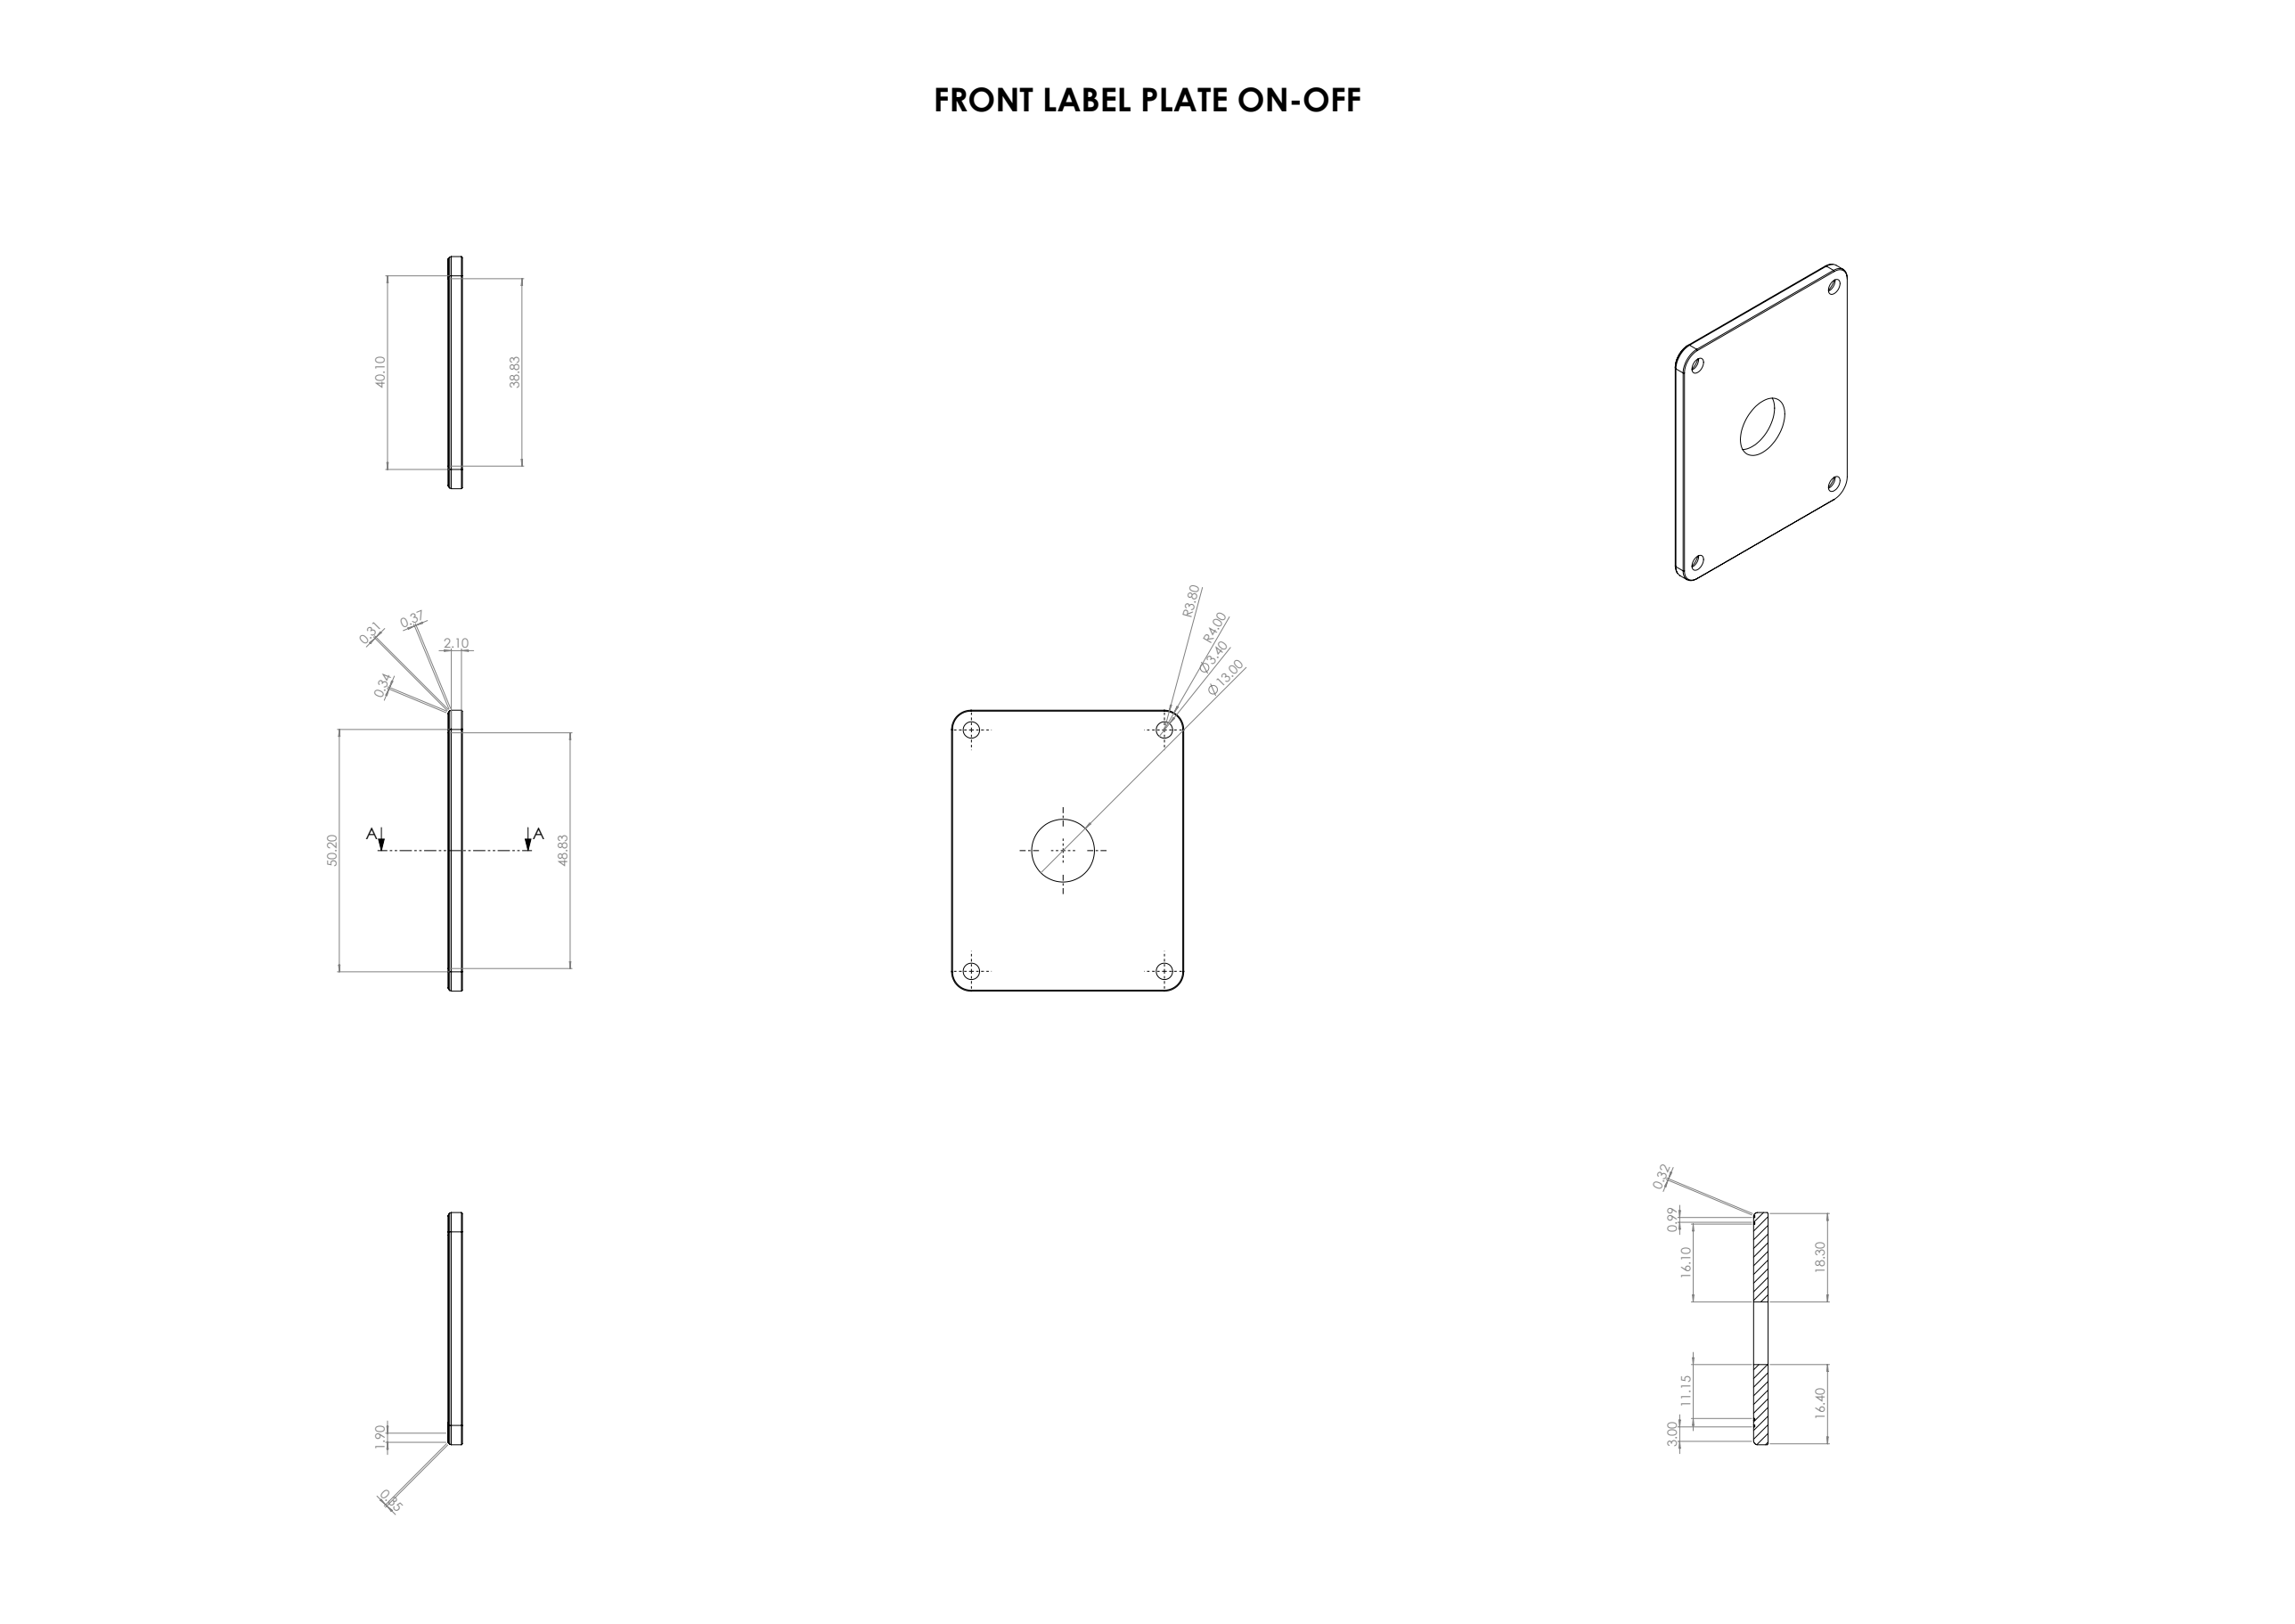
ISO-10303-21;
HEADER;
/* Generated by software containing ST-Developer
 * from STEP Tools, Inc. (www.steptools.com) 
 */

FILE_DESCRIPTION(
/* description */ (''),
/* implementation_level */ '2;1');

FILE_NAME(
/* name */ '06_Front_Label_Plate_ON-OFF.step',
/* time_stamp */ '2026-10-21T01:59:45-07:00',
/* author */ (''),
/* organization */ (''),
/* preprocessor_version */ 'ST-DEVELOPER v20.2',
/* originating_system */ 'Autodesk Translation Framework v15.15.0.0',
/* authorisation */ '');

FILE_SCHEMA (('AUTOMOTIVE_DESIGN { 1 0 10303 214 3 1 1 }'));
ENDSEC;

DATA;
#10=MECHANICAL_DESIGN_GEOMETRIC_PRESENTATION_REPRESENTATION('',(#465),#18281);
#107=(
BOUNDED_CURVE()
B_SPLINE_CURVE(2,(#12695,#12696,#12697),.UNSPECIFIED.,.F.,.F.)
B_SPLINE_CURVE_WITH_KNOTS((3,3),(0.,0.110982483350979),.UNSPECIFIED.)
CURVE()
GEOMETRIC_REPRESENTATION_ITEM()
RATIONAL_B_SPLINE_CURVE((1.,1.,1.))
REPRESENTATION_ITEM('')
);
#108=(
BOUNDED_CURVE()
B_SPLINE_CURVE(2,(#12710,#12711,#12712),.UNSPECIFIED.,.F.,.F.)
B_SPLINE_CURVE_WITH_KNOTS((3,3),(0.058586025044114,0.117172050088227),
 .UNSPECIFIED.)
CURVE()
GEOMETRIC_REPRESENTATION_ITEM()
RATIONAL_B_SPLINE_CURVE((1.,1.,1.))
REPRESENTATION_ITEM('')
);
#109=(
BOUNDED_CURVE()
B_SPLINE_CURVE(2,(#12739,#12740,#12741),.UNSPECIFIED.,.F.,.F.)
B_SPLINE_CURVE_WITH_KNOTS((3,3),(0.,0.0585860250441136),.UNSPECIFIED.)
CURVE()
GEOMETRIC_REPRESENTATION_ITEM()
RATIONAL_B_SPLINE_CURVE((1.,1.,1.))
REPRESENTATION_ITEM('')
);
#110=(
BOUNDED_CURVE()
B_SPLINE_CURVE(2,(#12754,#12755,#12756),.UNSPECIFIED.,.F.,.F.)
B_SPLINE_CURVE_WITH_KNOTS((3,3),(0.0909175021833372,0.201899986183551),
 .UNSPECIFIED.)
CURVE()
GEOMETRIC_REPRESENTATION_ITEM()
RATIONAL_B_SPLINE_CURVE((1.,1.,1.))
REPRESENTATION_ITEM('')
);
#111=(
BOUNDED_CURVE()
B_SPLINE_CURVE(2,(#12765,#12766,#12767),.UNSPECIFIED.,.F.,.F.)
B_SPLINE_CURVE_WITH_KNOTS((3,3),(0.0485753412182672,0.117172050088219),
 .UNSPECIFIED.)
CURVE()
GEOMETRIC_REPRESENTATION_ITEM()
RATIONAL_B_SPLINE_CURVE((1.,1.,1.))
REPRESENTATION_ITEM('')
);
#112=(
BOUNDED_CURVE()
B_SPLINE_CURVE(2,(#12779,#12780,#12781),.UNSPECIFIED.,.F.,.F.)
B_SPLINE_CURVE_WITH_KNOTS((3,3),(0.0585860250445827,0.117172050088221),
 .UNSPECIFIED.)
CURVE()
GEOMETRIC_REPRESENTATION_ITEM()
RATIONAL_B_SPLINE_CURVE((1.,1.,1.))
REPRESENTATION_ITEM('')
);
#113=(
BOUNDED_CURVE()
B_SPLINE_CURVE(2,(#12785,#12786,#12787),.UNSPECIFIED.,.F.,.F.)
B_SPLINE_CURVE_WITH_KNOTS((3,3),(0.,0.068596708869952),.UNSPECIFIED.)
CURVE()
GEOMETRIC_REPRESENTATION_ITEM()
RATIONAL_B_SPLINE_CURVE((1.,1.,1.))
REPRESENTATION_ITEM('')
);
#114=(
BOUNDED_CURVE()
B_SPLINE_CURVE(2,(#12799,#12800,#12801),.UNSPECIFIED.,.F.,.F.)
B_SPLINE_CURVE_WITH_KNOTS((3,3),(0.0485753412182676,0.0585860250445827),
 .UNSPECIFIED.)
CURVE()
GEOMETRIC_REPRESENTATION_ITEM()
RATIONAL_B_SPLINE_CURVE((1.,1.,1.))
REPRESENTATION_ITEM('')
);
#115=(
BOUNDED_CURVE()
B_SPLINE_CURVE(2,(#13088,#13089,#13090),.UNSPECIFIED.,.F.,.F.)
B_SPLINE_CURVE_WITH_KNOTS((3,3),(0.058586025043638,0.0685967088699541),
 .UNSPECIFIED.)
CURVE()
GEOMETRIC_REPRESENTATION_ITEM()
RATIONAL_B_SPLINE_CURVE((1.,1.,1.))
REPRESENTATION_ITEM('')
);
#116=(
BOUNDED_CURVE()
B_SPLINE_CURVE(2,(#13101,#13102,#13103),.UNSPECIFIED.,.F.,.F.)
B_SPLINE_CURVE_WITH_KNOTS((3,3),(0.,0.058586025043638),.UNSPECIFIED.)
CURVE()
GEOMETRIC_REPRESENTATION_ITEM()
RATIONAL_B_SPLINE_CURVE((1.,1.,1.))
REPRESENTATION_ITEM('')
);
#143=B_SPLINE_SURFACE_WITH_KNOTS('',2,1,((#12638,#12639),(#12640,#12641),
(#12642,#12643),(#12644,#12645),(#12646,#12647),(#12648,#12649),(#12650,
#12651)),.UNSPECIFIED.,.F.,.F.,.F.,(3,2,2,3),(2,2),(-1.09408743911249,0.,
1.,1.84668421503224),(-0.0908822509939087,0.140882250993909),
 .UNSPECIFIED.);
#144=B_SPLINE_SURFACE_WITH_KNOTS('',2,1,((#13225,#13226),(#13227,#13228),
(#13229,#13230),(#13231,#13232),(#13233,#13234),(#13235,#13236),(#13237,
#13238)),.UNSPECIFIED.,.F.,.F.,.F.,(3,2,2,3),(2,2),(-0.763868143299771,
0.,1.,1.96021762995607),(-0.090882250993909,0.140882250993909),
 .UNSPECIFIED.);
#145=B_SPLINE_SURFACE_WITH_KNOTS('',2,1,((#13240,#13241),(#13242,#13243),
(#13244,#13245)),.UNSPECIFIED.,.F.,.F.,.F.,(3,3),(2,2),(0.,1.),(0.,0.025),
 .UNSPECIFIED.);
#146=B_SPLINE_SURFACE_WITH_KNOTS('',2,1,((#13247,#13248),(#13249,#13250),
(#13251,#13252)),.UNSPECIFIED.,.F.,.F.,.F.,(3,3),(2,2),(0.,1.),(0.,0.025),
 .UNSPECIFIED.);
#147=B_SPLINE_SURFACE_WITH_KNOTS('',2,1,((#13254,#13255),(#13256,#13257),
(#13258,#13259)),.UNSPECIFIED.,.F.,.F.,.F.,(3,3),(2,2),(0.,1.),(0.,0.025),
 .UNSPECIFIED.);
#148=B_SPLINE_SURFACE_WITH_KNOTS('',2,1,((#13261,#13262),(#13263,#13264),
(#13265,#13266)),.UNSPECIFIED.,.F.,.F.,.F.,(3,3),(2,2),(0.,1.),(0.,0.025),
 .UNSPECIFIED.);
#149=B_SPLINE_SURFACE_WITH_KNOTS('',2,1,((#13268,#13269),(#13270,#13271),
(#13272,#13273)),.UNSPECIFIED.,.F.,.F.,.F.,(3,3),(2,2),(0.,1.),(0.,0.025),
 .UNSPECIFIED.);
#150=B_SPLINE_SURFACE_WITH_KNOTS('',2,1,((#13356,#13357),(#13358,#13359),
(#13360,#13361)),.UNSPECIFIED.,.F.,.F.,.F.,(3,3),(2,2),(0.,1.),(0.,0.025),
 .UNSPECIFIED.);
#151=B_SPLINE_SURFACE_WITH_KNOTS('',2,1,((#13369,#13370),(#13371,#13372),
(#13373,#13374)),.UNSPECIFIED.,.F.,.F.,.F.,(3,3),(2,2),(0.,1.),(0.,0.025),
 .UNSPECIFIED.);
#152=B_SPLINE_SURFACE_WITH_KNOTS('',2,1,((#13380,#13381),(#13382,#13383),
(#13384,#13385)),.UNSPECIFIED.,.F.,.F.,.F.,(3,3),(2,2),(0.,1.),(0.,0.025),
 .UNSPECIFIED.);
#153=B_SPLINE_SURFACE_WITH_KNOTS('',2,1,((#13391,#13392),(#13393,#13394),
(#13395,#13396)),.UNSPECIFIED.,.F.,.F.,.F.,(3,3),(2,2),(0.,1.),(0.,0.025),
 .UNSPECIFIED.);
#154=B_SPLINE_SURFACE_WITH_KNOTS('',2,1,((#13402,#13403),(#13404,#13405),
(#13406,#13407)),.UNSPECIFIED.,.F.,.F.,.F.,(3,3),(2,2),(0.,1.),(0.,0.025),
 .UNSPECIFIED.);
#155=B_SPLINE_SURFACE_WITH_KNOTS('',2,1,((#13413,#13414),(#13415,#13416),
(#13417,#13418)),.UNSPECIFIED.,.F.,.F.,.F.,(3,3),(2,2),(0.,1.),(0.,0.025),
 .UNSPECIFIED.);
#156=B_SPLINE_SURFACE_WITH_KNOTS('',2,1,((#13424,#13425),(#13426,#13427),
(#13428,#13429)),.UNSPECIFIED.,.F.,.F.,.F.,(3,3),(2,2),(0.,1.),(0.,0.025),
 .UNSPECIFIED.);
#157=B_SPLINE_SURFACE_WITH_KNOTS('',2,1,((#13435,#13436),(#13437,#13438),
(#13439,#13440)),.UNSPECIFIED.,.F.,.F.,.F.,(3,3),(2,2),(0.,1.),(0.,0.025),
 .UNSPECIFIED.);
#158=B_SPLINE_SURFACE_WITH_KNOTS('',2,1,((#13446,#13447),(#13448,#13449),
(#13450,#13451)),.UNSPECIFIED.,.F.,.F.,.F.,(3,3),(2,2),(0.,1.),(0.,0.025),
 .UNSPECIFIED.);
#159=B_SPLINE_SURFACE_WITH_KNOTS('',2,1,((#13457,#13458),(#13459,#13460),
(#13461,#13462)),.UNSPECIFIED.,.F.,.F.,.F.,(3,3),(2,2),(0.,1.),(0.,0.025),
 .UNSPECIFIED.);
#160=B_SPLINE_SURFACE_WITH_KNOTS('',2,1,((#13468,#13469),(#13470,#13471),
(#13472,#13473)),.UNSPECIFIED.,.F.,.F.,.F.,(3,3),(2,2),(0.,1.),(0.,0.025),
 .UNSPECIFIED.);
#161=B_SPLINE_SURFACE_WITH_KNOTS('',2,1,((#13519,#13520),(#13521,#13522),
(#13523,#13524)),.UNSPECIFIED.,.F.,.F.,.F.,(3,3),(2,2),(0.,1.),(0.,0.025),
 .UNSPECIFIED.);
#162=B_SPLINE_SURFACE_WITH_KNOTS('',2,1,((#13532,#13533),(#13534,#13535),
(#13536,#13537)),.UNSPECIFIED.,.F.,.F.,.F.,(3,3),(2,2),(0.,1.),(0.,0.025),
 .UNSPECIFIED.);
#163=B_SPLINE_SURFACE_WITH_KNOTS('',2,1,((#13543,#13544),(#13545,#13546),
(#13547,#13548)),.UNSPECIFIED.,.F.,.F.,.F.,(3,3),(2,2),(0.,1.),(0.,0.025),
 .UNSPECIFIED.);
#164=B_SPLINE_SURFACE_WITH_KNOTS('',2,1,((#13554,#13555),(#13556,#13557),
(#13558,#13559)),.UNSPECIFIED.,.F.,.F.,.F.,(3,3),(2,2),(0.,1.),(0.,0.025),
 .UNSPECIFIED.);
#165=B_SPLINE_SURFACE_WITH_KNOTS('',2,1,((#13565,#13566),(#13567,#13568),
(#13569,#13570)),.UNSPECIFIED.,.F.,.F.,.F.,(3,3),(2,2),(0.,1.),(0.,0.025),
 .UNSPECIFIED.);
#166=B_SPLINE_SURFACE_WITH_KNOTS('',2,1,((#13576,#13577),(#13578,#13579),
(#13580,#13581)),.UNSPECIFIED.,.F.,.F.,.F.,(3,3),(2,2),(0.,1.),(0.,0.025),
 .UNSPECIFIED.);
#167=B_SPLINE_SURFACE_WITH_KNOTS('',2,1,((#13587,#13588),(#13589,#13590),
(#13591,#13592)),.UNSPECIFIED.,.F.,.F.,.F.,(3,3),(2,2),(0.,1.),(0.,0.025),
 .UNSPECIFIED.);
#168=B_SPLINE_SURFACE_WITH_KNOTS('',2,1,((#13598,#13599),(#13600,#13601),
(#13602,#13603)),.UNSPECIFIED.,.F.,.F.,.F.,(3,3),(2,2),(0.,1.),(0.,0.025),
 .UNSPECIFIED.);
#169=B_SPLINE_SURFACE_WITH_KNOTS('',2,1,((#13609,#13610),(#13611,#13612),
(#13613,#13614)),.UNSPECIFIED.,.F.,.F.,.F.,(3,3),(2,2),(0.,1.),(0.,0.025),
 .UNSPECIFIED.);
#170=B_SPLINE_SURFACE_WITH_KNOTS('',2,1,((#13620,#13621),(#13622,#13623),
(#13624,#13625)),.UNSPECIFIED.,.F.,.F.,.F.,(3,3),(2,2),(0.,1.),(0.,0.025),
 .UNSPECIFIED.);
#171=B_SPLINE_SURFACE_WITH_KNOTS('',2,1,((#13631,#13632),(#13633,#13634),
(#13635,#13636)),.UNSPECIFIED.,.F.,.F.,.F.,(3,3),(2,2),(0.,1.),(0.,0.025),
 .UNSPECIFIED.);
#172=B_SPLINE_SURFACE_WITH_KNOTS('',2,1,((#13682,#13683),(#13684,#13685),
(#13686,#13687)),.UNSPECIFIED.,.F.,.F.,.F.,(3,3),(2,2),(0.,1.),(0.,0.025),
 .UNSPECIFIED.);
#173=B_SPLINE_SURFACE_WITH_KNOTS('',2,1,((#13695,#13696),(#13697,#13698),
(#13699,#13700)),.UNSPECIFIED.,.F.,.F.,.F.,(3,3),(2,2),(0.,1.),(0.,0.025),
 .UNSPECIFIED.);
#174=B_SPLINE_SURFACE_WITH_KNOTS('',2,1,((#13706,#13707),(#13708,#13709),
(#13710,#13711)),.UNSPECIFIED.,.F.,.F.,.F.,(3,3),(2,2),(0.,1.),(0.,0.025),
 .UNSPECIFIED.);
#175=B_SPLINE_SURFACE_WITH_KNOTS('',2,1,((#13717,#13718),(#13719,#13720),
(#13721,#13722)),.UNSPECIFIED.,.F.,.F.,.F.,(3,3),(2,2),(0.,1.),(0.,0.025),
 .UNSPECIFIED.);
#176=B_SPLINE_SURFACE_WITH_KNOTS('',2,1,((#13728,#13729),(#13730,#13731),
(#13732,#13733)),.UNSPECIFIED.,.F.,.F.,.F.,(3,3),(2,2),(0.,1.),(0.,0.025),
 .UNSPECIFIED.);
#177=B_SPLINE_SURFACE_WITH_KNOTS('',2,1,((#13739,#13740),(#13741,#13742),
(#13743,#13744)),.UNSPECIFIED.,.F.,.F.,.F.,(3,3),(2,2),(0.,1.),(0.,0.025),
 .UNSPECIFIED.);
#178=B_SPLINE_SURFACE_WITH_KNOTS('',2,1,((#13750,#13751),(#13752,#13753),
(#13754,#13755)),.UNSPECIFIED.,.F.,.F.,.F.,(3,3),(2,2),(0.,1.),(0.,0.025),
 .UNSPECIFIED.);
#179=B_SPLINE_SURFACE_WITH_KNOTS('',2,1,((#13761,#13762),(#13763,#13764),
(#13765,#13766)),.UNSPECIFIED.,.F.,.F.,.F.,(3,3),(2,2),(0.,1.),(0.,0.025),
 .UNSPECIFIED.);
#180=B_SPLINE_SURFACE_WITH_KNOTS('',2,1,((#13772,#13773),(#13774,#13775),
(#13776,#13777)),.UNSPECIFIED.,.F.,.F.,.F.,(3,3),(2,2),(0.,1.),(0.,0.025),
 .UNSPECIFIED.);
#181=B_SPLINE_SURFACE_WITH_KNOTS('',2,1,((#13783,#13784),(#13785,#13786),
(#13787,#13788)),.UNSPECIFIED.,.F.,.F.,.F.,(3,3),(2,2),(0.,1.),(0.,0.025),
 .UNSPECIFIED.);
#182=B_SPLINE_SURFACE_WITH_KNOTS('',2,1,((#13794,#13795),(#13796,#13797),
(#13798,#13799)),.UNSPECIFIED.,.F.,.F.,.F.,(3,3),(2,2),(0.,1.),(0.,0.025),
 .UNSPECIFIED.);
#188=B_SPLINE_CURVE_WITH_KNOTS('',3,(#12551,#12552,#12553,#12554),
 .UNSPECIFIED.,.F.,.F.,(4,4),(-0.0416286806186443,-0.039090786429231),
 .UNSPECIFIED.);
#189=B_SPLINE_CURVE_WITH_KNOTS('',3,(#12563,#12564,#12565,#12566),
 .UNSPECIFIED.,.F.,.F.,(4,4),(-0.00358674747543116,-0.00105074276589837),
 .UNSPECIFIED.);
#190=B_SPLINE_CURVE_WITH_KNOTS('',3,(#12609,#12610,#12611,#12612,#12613,
#12614,#12615),.UNSPECIFIED.,.F.,.F.,(4,3,4),(0.,0.0165311745375961,0.035733654742842),
 .UNSPECIFIED.);
#191=B_SPLINE_CURVE_WITH_KNOTS('',3,(#12616,#12617,#12618,#12619,#12620,
#12621,#12622),.UNSPECIFIED.,.F.,.F.,(4,3,4),(0.093322390013544,0.111401256244007,
0.119257131462378),.UNSPECIFIED.);
#192=B_SPLINE_CURVE_WITH_KNOTS('',3,(#12625,#12626,#12627,#12628,#12629,
#12630,#12631),.UNSPECIFIED.,.F.,.F.,(4,3,4),(0.107846162587432,0.120934849613304,
0.1266096642358),.UNSPECIFIED.);
#193=B_SPLINE_CURVE_WITH_KNOTS('',3,(#12633,#12634,#12635,#12636),
 .UNSPECIFIED.,.F.,.F.,(4,4),(0.,0.0156100092084493),.UNSPECIFIED.);
#194=B_SPLINE_CURVE_WITH_KNOTS('',3,(#12653,#12654,#12655,#12656),
 .UNSPECIFIED.,.F.,.F.,(4,4),(-0.159704010702857,-0.0871316914258202),
 .UNSPECIFIED.);
#195=B_SPLINE_CURVE_WITH_KNOTS('',2,(#12658,#12659,#12660),
 .UNSPECIFIED.,.F.,.F.,(3,3),(0.626600308945203,1.),.UNSPECIFIED.);
#196=B_SPLINE_CURVE_WITH_KNOTS('',2,(#12664,#12665,#12666),
 .UNSPECIFIED.,.F.,.F.,(3,3),(0.930285828630975,1.),.UNSPECIFIED.);
#197=B_SPLINE_CURVE_WITH_KNOTS('',3,(#12667,#12668,#12669,#12670,#12671,
#12672,#12673),.UNSPECIFIED.,.F.,.F.,(4,3,4),(-0.0373027797814653,-0.0240644534710859,
0.),.UNSPECIFIED.);
#198=B_SPLINE_CURVE_WITH_KNOTS('',3,(#12676,#12677,#12678,#12679,#12680,
#12681,#12682,#12683,#12684,#12685),.UNSPECIFIED.,.F.,.F.,(4,3,3,4),(-0.19290526608905,
-0.149564698200622,-0.106837983631372,-0.0956446006455143),
 .UNSPECIFIED.);
#199=B_SPLINE_CURVE_WITH_KNOTS('',3,(#12699,#12700,#12701,#12702,#12703,
#12704,#12705,#12706,#12707,#12708),.UNSPECIFIED.,.F.,.F.,(4,2,2,2,4),(0.00995060155970214,
0.127861262644591,0.255722525289182,0.384625287958343,0.513528050627505),
 .UNSPECIFIED.);
#200=B_SPLINE_CURVE_WITH_KNOTS('',3,(#12743,#12744,#12745,#12746,#12747,
#12748,#12749,#12750,#12751,#12752),.UNSPECIFIED.,.F.,.F.,(4,2,2,2,4),(1.52050309692962,
1.64940585959878,1.77830862226794,1.90616988491253,2.02408054599742),
 .UNSPECIFIED.);
#201=B_SPLINE_CURVE_WITH_KNOTS('',3,(#12789,#12790,#12791,#12792,#12793,
#12794,#12795,#12796,#12797,#12798),.UNSPECIFIED.,.F.,.F.,(4,2,2,2,4),(0.518398684879072,
0.638089519791373,0.767732342509753,0.897375165228133,1.01706600014044),
 .UNSPECIFIED.);
#202=B_SPLINE_CURVE_WITH_KNOTS('',2,(#12813,#12814,#12815),
 .UNSPECIFIED.,.F.,.F.,(3,3),(0.,1.),.UNSPECIFIED.);
#203=B_SPLINE_CURVE_WITH_KNOTS('',2,(#12817,#12818,#12819),
 .UNSPECIFIED.,.F.,.F.,(3,3),(0.,1.),.UNSPECIFIED.);
#204=B_SPLINE_CURVE_WITH_KNOTS('',2,(#12821,#12822,#12823),
 .UNSPECIFIED.,.F.,.F.,(3,3),(0.,1.),.UNSPECIFIED.);
#205=B_SPLINE_CURVE_WITH_KNOTS('',2,(#12825,#12826,#12827),
 .UNSPECIFIED.,.F.,.F.,(3,3),(0.,1.),.UNSPECIFIED.);
#206=B_SPLINE_CURVE_WITH_KNOTS('',2,(#12829,#12830,#12831),
 .UNSPECIFIED.,.F.,.F.,(3,3),(0.,1.),.UNSPECIFIED.);
#207=B_SPLINE_CURVE_WITH_KNOTS('',2,(#12832,#12833,#12834),
 .UNSPECIFIED.,.F.,.F.,(3,3),(0.,0.31406597767443),.UNSPECIFIED.);
#208=B_SPLINE_CURVE_WITH_KNOTS('',2,(#12906,#12907,#12908),
 .UNSPECIFIED.,.F.,.F.,(3,3),(0.,1.),.UNSPECIFIED.);
#209=B_SPLINE_CURVE_WITH_KNOTS('',2,(#12910,#12911,#12912),
 .UNSPECIFIED.,.F.,.F.,(3,3),(0.,1.),.UNSPECIFIED.);
#210=B_SPLINE_CURVE_WITH_KNOTS('',2,(#12914,#12915,#12916),
 .UNSPECIFIED.,.F.,.F.,(3,3),(0.,1.),.UNSPECIFIED.);
#211=B_SPLINE_CURVE_WITH_KNOTS('',2,(#12918,#12919,#12920),
 .UNSPECIFIED.,.F.,.F.,(3,3),(0.,1.),.UNSPECIFIED.);
#212=B_SPLINE_CURVE_WITH_KNOTS('',2,(#12922,#12923,#12924),
 .UNSPECIFIED.,.F.,.F.,(3,3),(0.,1.),.UNSPECIFIED.);
#213=B_SPLINE_CURVE_WITH_KNOTS('',2,(#12926,#12927,#12928),
 .UNSPECIFIED.,.F.,.F.,(3,3),(0.,1.),.UNSPECIFIED.);
#214=B_SPLINE_CURVE_WITH_KNOTS('',2,(#12930,#12931,#12932),
 .UNSPECIFIED.,.F.,.F.,(3,3),(0.,1.),.UNSPECIFIED.);
#215=B_SPLINE_CURVE_WITH_KNOTS('',2,(#12934,#12935,#12936),
 .UNSPECIFIED.,.F.,.F.,(3,3),(0.,1.),.UNSPECIFIED.);
#216=B_SPLINE_CURVE_WITH_KNOTS('',2,(#12938,#12939,#12940),
 .UNSPECIFIED.,.F.,.F.,(3,3),(0.,1.),.UNSPECIFIED.);
#217=B_SPLINE_CURVE_WITH_KNOTS('',2,(#12942,#12943,#12944),
 .UNSPECIFIED.,.F.,.F.,(3,3),(0.,1.),.UNSPECIFIED.);
#218=B_SPLINE_CURVE_WITH_KNOTS('',2,(#12945,#12946,#12947),
 .UNSPECIFIED.,.F.,.F.,(3,3),(0.,1.),.UNSPECIFIED.);
#219=B_SPLINE_CURVE_WITH_KNOTS('',2,(#12970,#12971,#12972),
 .UNSPECIFIED.,.F.,.F.,(3,3),(0.,1.),.UNSPECIFIED.);
#220=B_SPLINE_CURVE_WITH_KNOTS('',2,(#12974,#12975,#12976),
 .UNSPECIFIED.,.F.,.F.,(3,3),(0.,1.),.UNSPECIFIED.);
#221=B_SPLINE_CURVE_WITH_KNOTS('',2,(#12978,#12979,#12980),
 .UNSPECIFIED.,.F.,.F.,(3,3),(0.,1.),.UNSPECIFIED.);
#222=B_SPLINE_CURVE_WITH_KNOTS('',2,(#12982,#12983,#12984),
 .UNSPECIFIED.,.F.,.F.,(3,3),(0.,1.),.UNSPECIFIED.);
#223=B_SPLINE_CURVE_WITH_KNOTS('',2,(#12986,#12987,#12988),
 .UNSPECIFIED.,.F.,.F.,(3,3),(0.,1.),.UNSPECIFIED.);
#224=B_SPLINE_CURVE_WITH_KNOTS('',2,(#12990,#12991,#12992),
 .UNSPECIFIED.,.F.,.F.,(3,3),(0.,1.),.UNSPECIFIED.);
#225=B_SPLINE_CURVE_WITH_KNOTS('',2,(#12994,#12995,#12996),
 .UNSPECIFIED.,.F.,.F.,(3,3),(0.,1.),.UNSPECIFIED.);
#226=B_SPLINE_CURVE_WITH_KNOTS('',2,(#12998,#12999,#13000),
 .UNSPECIFIED.,.F.,.F.,(3,3),(0.,1.),.UNSPECIFIED.);
#227=B_SPLINE_CURVE_WITH_KNOTS('',2,(#13002,#13003,#13004),
 .UNSPECIFIED.,.F.,.F.,(3,3),(0.,1.),.UNSPECIFIED.);
#228=B_SPLINE_CURVE_WITH_KNOTS('',2,(#13006,#13007,#13008),
 .UNSPECIFIED.,.F.,.F.,(3,3),(0.,1.),.UNSPECIFIED.);
#229=B_SPLINE_CURVE_WITH_KNOTS('',2,(#13009,#13010,#13011),
 .UNSPECIFIED.,.F.,.F.,(3,3),(0.,1.),.UNSPECIFIED.);
#230=B_SPLINE_CURVE_WITH_KNOTS('',2,(#13016,#13017,#13018),
 .UNSPECIFIED.,.F.,.F.,(3,3),(0.,1.),.UNSPECIFIED.);
#231=B_SPLINE_CURVE_WITH_KNOTS('',2,(#13020,#13021,#13022),
 .UNSPECIFIED.,.F.,.F.,(3,3),(0.,1.),.UNSPECIFIED.);
#232=B_SPLINE_CURVE_WITH_KNOTS('',2,(#13024,#13025,#13026),
 .UNSPECIFIED.,.F.,.F.,(3,3),(0.,1.),.UNSPECIFIED.);
#233=B_SPLINE_CURVE_WITH_KNOTS('',2,(#13028,#13029,#13030),
 .UNSPECIFIED.,.F.,.F.,(3,3),(0.,1.),.UNSPECIFIED.);
#234=B_SPLINE_CURVE_WITH_KNOTS('',2,(#13032,#13033,#13034),
 .UNSPECIFIED.,.F.,.F.,(3,3),(0.,1.),.UNSPECIFIED.);
#235=B_SPLINE_CURVE_WITH_KNOTS('',2,(#13036,#13037,#13038),
 .UNSPECIFIED.,.F.,.F.,(3,3),(0.,1.),.UNSPECIFIED.);
#236=B_SPLINE_CURVE_WITH_KNOTS('',2,(#13040,#13041,#13042),
 .UNSPECIFIED.,.F.,.F.,(3,3),(0.,1.),.UNSPECIFIED.);
#237=B_SPLINE_CURVE_WITH_KNOTS('',2,(#13044,#13045,#13046),
 .UNSPECIFIED.,.F.,.F.,(3,3),(0.,1.),.UNSPECIFIED.);
#238=B_SPLINE_CURVE_WITH_KNOTS('',2,(#13048,#13049,#13050),
 .UNSPECIFIED.,.F.,.F.,(3,3),(0.,1.),.UNSPECIFIED.);
#239=B_SPLINE_CURVE_WITH_KNOTS('',2,(#13052,#13053,#13054),
 .UNSPECIFIED.,.F.,.F.,(3,3),(0.,1.),.UNSPECIFIED.);
#240=B_SPLINE_CURVE_WITH_KNOTS('',2,(#13055,#13056,#13057),
 .UNSPECIFIED.,.F.,.F.,(3,3),(0.,1.),.UNSPECIFIED.);
#241=B_SPLINE_CURVE_WITH_KNOTS('',3,(#13091,#13092,#13093,#13094,#13095,
#13096,#13097,#13098,#13099,#13100),.UNSPECIFIED.,.F.,.F.,(4,2,2,2,4),(1.01688813186998,
1.13657896678228,1.26622178950066,1.39586461221904,1.51555544713135),
 .UNSPECIFIED.);
#242=B_SPLINE_CURVE_WITH_KNOTS('',2,(#13149,#13150,#13151),
 .UNSPECIFIED.,.F.,.F.,(3,3),(0.,0.369411589751801),.UNSPECIFIED.);
#243=B_SPLINE_CURVE_WITH_KNOTS('',2,(#13153,#13154,#13155),
 .UNSPECIFIED.,.F.,.F.,(3,3),(0.,1.),.UNSPECIFIED.);
#244=B_SPLINE_CURVE_WITH_KNOTS('',2,(#13157,#13158,#13159),
 .UNSPECIFIED.,.F.,.F.,(3,3),(0.,1.),.UNSPECIFIED.);
#245=B_SPLINE_CURVE_WITH_KNOTS('',2,(#13161,#13162,#13163),
 .UNSPECIFIED.,.F.,.F.,(3,3),(0.,1.),.UNSPECIFIED.);
#246=B_SPLINE_CURVE_WITH_KNOTS('',2,(#13165,#13166,#13167),
 .UNSPECIFIED.,.F.,.F.,(3,3),(0.,1.),.UNSPECIFIED.);
#247=B_SPLINE_CURVE_WITH_KNOTS('',2,(#13168,#13169,#13170),
 .UNSPECIFIED.,.F.,.F.,(3,3),(0.,1.),.UNSPECIFIED.);
#248=B_SPLINE_CURVE_WITH_KNOTS('',2,(#13365,#13366,#13367),
 .UNSPECIFIED.,.F.,.F.,(3,3),(0.,1.),.UNSPECIFIED.);
#249=B_SPLINE_CURVE_WITH_KNOTS('',2,(#13377,#13378,#13379),
 .UNSPECIFIED.,.F.,.F.,(3,3),(0.,1.),.UNSPECIFIED.);
#250=B_SPLINE_CURVE_WITH_KNOTS('',2,(#13388,#13389,#13390),
 .UNSPECIFIED.,.F.,.F.,(3,3),(0.,1.),.UNSPECIFIED.);
#251=B_SPLINE_CURVE_WITH_KNOTS('',2,(#13399,#13400,#13401),
 .UNSPECIFIED.,.F.,.F.,(3,3),(0.,1.),.UNSPECIFIED.);
#252=B_SPLINE_CURVE_WITH_KNOTS('',2,(#13410,#13411,#13412),
 .UNSPECIFIED.,.F.,.F.,(3,3),(0.,1.),.UNSPECIFIED.);
#253=B_SPLINE_CURVE_WITH_KNOTS('',2,(#13421,#13422,#13423),
 .UNSPECIFIED.,.F.,.F.,(3,3),(0.,1.),.UNSPECIFIED.);
#254=B_SPLINE_CURVE_WITH_KNOTS('',2,(#13432,#13433,#13434),
 .UNSPECIFIED.,.F.,.F.,(3,3),(0.,1.),.UNSPECIFIED.);
#255=B_SPLINE_CURVE_WITH_KNOTS('',2,(#13443,#13444,#13445),
 .UNSPECIFIED.,.F.,.F.,(3,3),(0.,1.),.UNSPECIFIED.);
#256=B_SPLINE_CURVE_WITH_KNOTS('',2,(#13454,#13455,#13456),
 .UNSPECIFIED.,.F.,.F.,(3,3),(0.,1.),.UNSPECIFIED.);
#257=B_SPLINE_CURVE_WITH_KNOTS('',2,(#13465,#13466,#13467),
 .UNSPECIFIED.,.F.,.F.,(3,3),(0.,1.),.UNSPECIFIED.);
#258=B_SPLINE_CURVE_WITH_KNOTS('',2,(#13474,#13475,#13476),
 .UNSPECIFIED.,.F.,.F.,(3,3),(0.,1.),.UNSPECIFIED.);
#259=B_SPLINE_CURVE_WITH_KNOTS('',2,(#13528,#13529,#13530),
 .UNSPECIFIED.,.F.,.F.,(3,3),(0.,1.),.UNSPECIFIED.);
#260=B_SPLINE_CURVE_WITH_KNOTS('',2,(#13540,#13541,#13542),
 .UNSPECIFIED.,.F.,.F.,(3,3),(0.,1.),.UNSPECIFIED.);
#261=B_SPLINE_CURVE_WITH_KNOTS('',2,(#13551,#13552,#13553),
 .UNSPECIFIED.,.F.,.F.,(3,3),(0.,1.),.UNSPECIFIED.);
#262=B_SPLINE_CURVE_WITH_KNOTS('',2,(#13562,#13563,#13564),
 .UNSPECIFIED.,.F.,.F.,(3,3),(0.,1.),.UNSPECIFIED.);
#263=B_SPLINE_CURVE_WITH_KNOTS('',2,(#13573,#13574,#13575),
 .UNSPECIFIED.,.F.,.F.,(3,3),(0.,1.),.UNSPECIFIED.);
#264=B_SPLINE_CURVE_WITH_KNOTS('',2,(#13584,#13585,#13586),
 .UNSPECIFIED.,.F.,.F.,(3,3),(0.,1.),.UNSPECIFIED.);
#265=B_SPLINE_CURVE_WITH_KNOTS('',2,(#13595,#13596,#13597),
 .UNSPECIFIED.,.F.,.F.,(3,3),(0.,1.),.UNSPECIFIED.);
#266=B_SPLINE_CURVE_WITH_KNOTS('',2,(#13606,#13607,#13608),
 .UNSPECIFIED.,.F.,.F.,(3,3),(0.,1.),.UNSPECIFIED.);
#267=B_SPLINE_CURVE_WITH_KNOTS('',2,(#13617,#13618,#13619),
 .UNSPECIFIED.,.F.,.F.,(3,3),(0.,1.),.UNSPECIFIED.);
#268=B_SPLINE_CURVE_WITH_KNOTS('',2,(#13628,#13629,#13630),
 .UNSPECIFIED.,.F.,.F.,(3,3),(0.,1.),.UNSPECIFIED.);
#269=B_SPLINE_CURVE_WITH_KNOTS('',2,(#13637,#13638,#13639),
 .UNSPECIFIED.,.F.,.F.,(3,3),(0.,1.),.UNSPECIFIED.);
#270=B_SPLINE_CURVE_WITH_KNOTS('',2,(#13691,#13692,#13693),
 .UNSPECIFIED.,.F.,.F.,(3,3),(0.,1.),.UNSPECIFIED.);
#271=B_SPLINE_CURVE_WITH_KNOTS('',2,(#13703,#13704,#13705),
 .UNSPECIFIED.,.F.,.F.,(3,3),(0.,1.),.UNSPECIFIED.);
#272=B_SPLINE_CURVE_WITH_KNOTS('',2,(#13714,#13715,#13716),
 .UNSPECIFIED.,.F.,.F.,(3,3),(0.,1.),.UNSPECIFIED.);
#273=B_SPLINE_CURVE_WITH_KNOTS('',2,(#13725,#13726,#13727),
 .UNSPECIFIED.,.F.,.F.,(3,3),(0.,1.),.UNSPECIFIED.);
#274=B_SPLINE_CURVE_WITH_KNOTS('',2,(#13736,#13737,#13738),
 .UNSPECIFIED.,.F.,.F.,(3,3),(0.,1.),.UNSPECIFIED.);
#275=B_SPLINE_CURVE_WITH_KNOTS('',2,(#13747,#13748,#13749),
 .UNSPECIFIED.,.F.,.F.,(3,3),(0.,1.),.UNSPECIFIED.);
#276=B_SPLINE_CURVE_WITH_KNOTS('',2,(#13758,#13759,#13760),
 .UNSPECIFIED.,.F.,.F.,(3,3),(0.,1.),.UNSPECIFIED.);
#277=B_SPLINE_CURVE_WITH_KNOTS('',2,(#13769,#13770,#13771),
 .UNSPECIFIED.,.F.,.F.,(3,3),(0.,1.),.UNSPECIFIED.);
#278=B_SPLINE_CURVE_WITH_KNOTS('',2,(#13780,#13781,#13782),
 .UNSPECIFIED.,.F.,.F.,(3,3),(0.,1.),.UNSPECIFIED.);
#279=B_SPLINE_CURVE_WITH_KNOTS('',2,(#13791,#13792,#13793),
 .UNSPECIFIED.,.F.,.F.,(3,3),(0.,1.),.UNSPECIFIED.);
#280=B_SPLINE_CURVE_WITH_KNOTS('',2,(#13800,#13801,#13802),
 .UNSPECIFIED.,.F.,.F.,(3,3),(0.,1.),.UNSPECIFIED.);
#368=CONICAL_SURFACE('',#9304,3.9,0.785398163397444);
#369=CONICAL_SURFACE('',#9308,3.9,0.785398163397444);
#370=CONICAL_SURFACE('',#9312,3.9,0.78539816339745);
#371=CONICAL_SURFACE('',#9316,3.9,0.78539816339745);
#372=CONICAL_SURFACE('',#9332,3.92928932188135,0.392699081698714);
#373=CONICAL_SURFACE('',#9335,3.92928932188135,0.392699081698714);
#374=CONICAL_SURFACE('',#9338,3.92928932188135,0.392699081698713);
#375=CONICAL_SURFACE('',#9342,3.92928932188135,0.392699081698724);
#376=CONICAL_SURFACE('',#9346,3.75,0.785398163397449);
#377=CONICAL_SURFACE('',#9349,3.75,0.785398163397447);
#378=CONICAL_SURFACE('',#9354,3.27928932188134,1.17809724509616);
#379=CONICAL_SURFACE('',#9358,3.47071067811865,1.17809724509617);
#380=CONICAL_SURFACE('',#9361,2.475,0.785398163397448);
#381=CONICAL_SURFACE('',#9363,3.27928932188134,1.17809724509616);
#382=CONICAL_SURFACE('',#9367,3.47071067811866,1.17809724509617);
#383=CONICAL_SURFACE('',#9369,2.475,0.785398163397448);
#384=CONICAL_SURFACE('',#9371,3.27928932188134,1.17809724509614);
#385=CONICAL_SURFACE('',#9378,2.475,0.785398163397449);
#386=CONICAL_SURFACE('',#9380,3.27928932188134,1.17809724509614);
#387=CONICAL_SURFACE('',#9382,2.475,0.785398163397449);
#388=CONICAL_SURFACE('',#9388,3.47071067811866,1.17809724509616);
#389=CONICAL_SURFACE('',#9390,3.47071067811866,1.17809724509616);
#390=CONICAL_SURFACE('',#9393,3.75,0.785398163397449);
#391=CONICAL_SURFACE('',#9395,3.75,0.785398163397449);
#439=SHAPE_REPRESENTATION_RELATIONSHIP('SRR','None',#18341,#452);
#452=ADVANCED_BREP_SHAPE_REPRESENTATION('',(#483),#18270);
#465=STYLED_ITEM('',(#18488),#483);
#483=MANIFOLD_SOLID_BREP('Body1',#9087);
#499=CYLINDRICAL_SURFACE('',#9319,4.);
#500=CYLINDRICAL_SURFACE('',#9322,4.);
#501=CYLINDRICAL_SURFACE('',#9462,1.7);
#502=CYLINDRICAL_SURFACE('',#9463,1.7);
#503=CYLINDRICAL_SURFACE('',#9464,1.7);
#504=CYLINDRICAL_SURFACE('',#9465,1.7);
#505=CYLINDRICAL_SURFACE('',#9466,6.5);
#506=CYLINDRICAL_SURFACE('',#9467,4.);
#507=CYLINDRICAL_SURFACE('',#9468,4.);
#585=FACE_BOUND('',#1422,.T.);
#586=FACE_BOUND('',#1423,.T.);
#587=FACE_BOUND('',#1424,.T.);
#588=FACE_BOUND('',#1425,.T.);
#589=FACE_BOUND('',#1426,.T.);
#590=FACE_BOUND('',#1454,.T.);
#591=FACE_BOUND('',#1455,.T.);
#592=FACE_BOUND('',#1456,.T.);
#593=FACE_BOUND('',#1457,.T.);
#594=FACE_BOUND('',#1458,.T.);
#595=FACE_BOUND('',#1459,.T.);
#596=FACE_BOUND('',#1460,.T.);
#597=FACE_BOUND('',#1461,.T.);
#639=CIRCLE('',#9305,4.);
#640=CIRCLE('',#9306,3.8);
#641=CIRCLE('',#9309,4.);
#642=CIRCLE('',#9310,3.8);
#643=CIRCLE('',#9313,4.);
#644=CIRCLE('',#9314,3.8);
#645=CIRCLE('',#9317,4.);
#646=CIRCLE('',#9318,3.8);
#647=CIRCLE('',#9320,4.);
#648=CIRCLE('',#9323,4.);
#649=CIRCLE('',#9326,1.7);
#650=CIRCLE('',#9327,1.7);
#651=CIRCLE('',#9328,1.7);
#652=CIRCLE('',#9329,1.7);
#653=CIRCLE('',#9330,6.5);
#654=CIRCLE('',#9333,3.85857864376269);
#655=CIRCLE('',#9336,3.85857864376269);
#656=CIRCLE('',#9339,3.85857864376269);
#657=CIRCLE('',#9340,4.);
#658=CIRCLE('',#9343,3.85857864376269);
#659=CIRCLE('',#9344,4.);
#660=CIRCLE('',#9347,3.64142135623731);
#661=CIRCLE('',#9350,3.64142135623731);
#662=CIRCLE('',#9355,3.10857864376269);
#663=CIRCLE('',#9356,3.45);
#664=CIRCLE('',#9357,3.45);
#665=CIRCLE('',#9359,3.64142135623731);
#666=CIRCLE('',#9362,1.7);
#667=CIRCLE('',#9364,3.10857864376269);
#668=CIRCLE('',#9365,3.45);
#669=CIRCLE('',#9366,3.45);
#670=CIRCLE('',#9370,1.7);
#671=CIRCLE('',#9372,3.1085786437627);
#672=CIRCLE('',#9373,3.44999999999999);
#673=CIRCLE('',#9376,3.44999999999999);
#674=CIRCLE('',#9377,6.5);
#675=CIRCLE('',#9379,1.7);
#676=CIRCLE('',#9381,3.1085786437627);
#677=CIRCLE('',#9383,1.7);
#678=CIRCLE('',#9391,3.64142135623731);
#881=FACE_OUTER_BOUND('',#1409,.T.);
#882=FACE_OUTER_BOUND('',#1410,.T.);
#883=FACE_OUTER_BOUND('',#1411,.T.);
#884=FACE_OUTER_BOUND('',#1412,.T.);
#885=FACE_OUTER_BOUND('',#1413,.T.);
#886=FACE_OUTER_BOUND('',#1414,.T.);
#887=FACE_OUTER_BOUND('',#1415,.T.);
#888=FACE_OUTER_BOUND('',#1416,.T.);
#889=FACE_OUTER_BOUND('',#1417,.T.);
#890=FACE_OUTER_BOUND('',#1418,.T.);
#891=FACE_OUTER_BOUND('',#1419,.T.);
#892=FACE_OUTER_BOUND('',#1420,.T.);
#893=FACE_OUTER_BOUND('',#1421,.T.);
#894=FACE_OUTER_BOUND('',#1427,.T.);
#895=FACE_OUTER_BOUND('',#1428,.T.);
#896=FACE_OUTER_BOUND('',#1429,.T.);
#897=FACE_OUTER_BOUND('',#1430,.T.);
#898=FACE_OUTER_BOUND('',#1431,.T.);
#899=FACE_OUTER_BOUND('',#1432,.T.);
#900=FACE_OUTER_BOUND('',#1433,.T.);
#901=FACE_OUTER_BOUND('',#1434,.T.);
#902=FACE_OUTER_BOUND('',#1435,.T.);
#903=FACE_OUTER_BOUND('',#1436,.T.);
#904=FACE_OUTER_BOUND('',#1437,.T.);
#905=FACE_OUTER_BOUND('',#1438,.T.);
#906=FACE_OUTER_BOUND('',#1439,.T.);
#907=FACE_OUTER_BOUND('',#1440,.T.);
#908=FACE_OUTER_BOUND('',#1441,.T.);
#909=FACE_OUTER_BOUND('',#1442,.T.);
#910=FACE_OUTER_BOUND('',#1443,.T.);
#911=FACE_OUTER_BOUND('',#1444,.T.);
#912=FACE_OUTER_BOUND('',#1445,.T.);
#913=FACE_OUTER_BOUND('',#1446,.T.);
#914=FACE_OUTER_BOUND('',#1447,.T.);
#915=FACE_OUTER_BOUND('',#1448,.T.);
#916=FACE_OUTER_BOUND('',#1449,.T.);
#917=FACE_OUTER_BOUND('',#1450,.T.);
#918=FACE_OUTER_BOUND('',#1451,.T.);
#919=FACE_OUTER_BOUND('',#1452,.T.);
#920=FACE_OUTER_BOUND('',#1453,.T.);
#921=FACE_OUTER_BOUND('',#1462,.T.);
#922=FACE_OUTER_BOUND('',#1463,.T.);
#923=FACE_OUTER_BOUND('',#1464,.T.);
#924=FACE_OUTER_BOUND('',#1465,.T.);
#925=FACE_OUTER_BOUND('',#1466,.T.);
#926=FACE_OUTER_BOUND('',#1467,.T.);
#927=FACE_OUTER_BOUND('',#1468,.T.);
#928=FACE_OUTER_BOUND('',#1469,.T.);
#929=FACE_OUTER_BOUND('',#1470,.T.);
#930=FACE_OUTER_BOUND('',#1471,.T.);
#931=FACE_OUTER_BOUND('',#1472,.T.);
#932=FACE_OUTER_BOUND('',#1473,.T.);
#933=FACE_OUTER_BOUND('',#1474,.T.);
#934=FACE_OUTER_BOUND('',#1475,.T.);
#935=FACE_OUTER_BOUND('',#1476,.T.);
#936=FACE_OUTER_BOUND('',#1477,.T.);
#937=FACE_OUTER_BOUND('',#1478,.T.);
#938=FACE_OUTER_BOUND('',#1479,.T.);
#939=FACE_OUTER_BOUND('',#1480,.T.);
#940=FACE_OUTER_BOUND('',#1481,.T.);
#941=FACE_OUTER_BOUND('',#1482,.T.);
#942=FACE_OUTER_BOUND('',#1483,.T.);
#943=FACE_OUTER_BOUND('',#1484,.T.);
#944=FACE_OUTER_BOUND('',#1485,.T.);
#945=FACE_OUTER_BOUND('',#1486,.T.);
#946=FACE_OUTER_BOUND('',#1487,.T.);
#947=FACE_OUTER_BOUND('',#1488,.T.);
#948=FACE_OUTER_BOUND('',#1489,.T.);
#949=FACE_OUTER_BOUND('',#1490,.T.);
#950=FACE_OUTER_BOUND('',#1491,.T.);
#951=FACE_OUTER_BOUND('',#1492,.T.);
#952=FACE_OUTER_BOUND('',#1493,.T.);
#953=FACE_OUTER_BOUND('',#1494,.T.);
#954=FACE_OUTER_BOUND('',#1495,.T.);
#955=FACE_OUTER_BOUND('',#1496,.T.);
#956=FACE_OUTER_BOUND('',#1497,.T.);
#957=FACE_OUTER_BOUND('',#1498,.T.);
#958=FACE_OUTER_BOUND('',#1499,.T.);
#959=FACE_OUTER_BOUND('',#1500,.T.);
#960=FACE_OUTER_BOUND('',#1501,.T.);
#961=FACE_OUTER_BOUND('',#1502,.T.);
#962=FACE_OUTER_BOUND('',#1503,.T.);
#963=FACE_OUTER_BOUND('',#1504,.T.);
#964=FACE_OUTER_BOUND('',#1505,.T.);
#965=FACE_OUTER_BOUND('',#1506,.T.);
#966=FACE_OUTER_BOUND('',#1507,.T.);
#967=FACE_OUTER_BOUND('',#1508,.T.);
#968=FACE_OUTER_BOUND('',#1509,.T.);
#969=FACE_OUTER_BOUND('',#1510,.T.);
#970=FACE_OUTER_BOUND('',#1511,.T.);
#971=FACE_OUTER_BOUND('',#1512,.T.);
#972=FACE_OUTER_BOUND('',#1513,.T.);
#973=FACE_OUTER_BOUND('',#1514,.T.);
#974=FACE_OUTER_BOUND('',#1515,.T.);
#975=FACE_OUTER_BOUND('',#1516,.T.);
#976=FACE_OUTER_BOUND('',#1517,.T.);
#977=FACE_OUTER_BOUND('',#1518,.T.);
#978=FACE_OUTER_BOUND('',#1519,.T.);
#979=FACE_OUTER_BOUND('',#1520,.T.);
#980=FACE_OUTER_BOUND('',#1521,.T.);
#981=FACE_OUTER_BOUND('',#1522,.T.);
#982=FACE_OUTER_BOUND('',#1523,.T.);
#983=FACE_OUTER_BOUND('',#1524,.T.);
#984=FACE_OUTER_BOUND('',#1525,.T.);
#985=FACE_OUTER_BOUND('',#1526,.T.);
#986=FACE_OUTER_BOUND('',#1527,.T.);
#987=FACE_OUTER_BOUND('',#1528,.T.);
#988=FACE_OUTER_BOUND('',#1529,.T.);
#989=FACE_OUTER_BOUND('',#1530,.T.);
#990=FACE_OUTER_BOUND('',#1531,.T.);
#991=FACE_OUTER_BOUND('',#1532,.T.);
#992=FACE_OUTER_BOUND('',#1533,.T.);
#993=FACE_OUTER_BOUND('',#1534,.T.);
#994=FACE_OUTER_BOUND('',#1535,.T.);
#995=FACE_OUTER_BOUND('',#1536,.T.);
#996=FACE_OUTER_BOUND('',#1537,.T.);
#997=FACE_OUTER_BOUND('',#1538,.T.);
#998=FACE_OUTER_BOUND('',#1539,.T.);
#999=FACE_OUTER_BOUND('',#1540,.T.);
#1000=FACE_OUTER_BOUND('',#1541,.T.);
#1001=FACE_OUTER_BOUND('',#1542,.T.);
#1002=FACE_OUTER_BOUND('',#1543,.T.);
#1003=FACE_OUTER_BOUND('',#1544,.T.);
#1004=FACE_OUTER_BOUND('',#1545,.T.);
#1005=FACE_OUTER_BOUND('',#1546,.T.);
#1006=FACE_OUTER_BOUND('',#1547,.T.);
#1007=FACE_OUTER_BOUND('',#1548,.T.);
#1008=FACE_OUTER_BOUND('',#1549,.T.);
#1009=FACE_OUTER_BOUND('',#1550,.T.);
#1010=FACE_OUTER_BOUND('',#1551,.T.);
#1011=FACE_OUTER_BOUND('',#1552,.T.);
#1012=FACE_OUTER_BOUND('',#1553,.T.);
#1013=FACE_OUTER_BOUND('',#1554,.T.);
#1014=FACE_OUTER_BOUND('',#1555,.T.);
#1015=FACE_OUTER_BOUND('',#1556,.T.);
#1016=FACE_OUTER_BOUND('',#1557,.T.);
#1017=FACE_OUTER_BOUND('',#1558,.T.);
#1018=FACE_OUTER_BOUND('',#1559,.T.);
#1019=FACE_OUTER_BOUND('',#1560,.T.);
#1020=FACE_OUTER_BOUND('',#1561,.T.);
#1021=FACE_OUTER_BOUND('',#1562,.T.);
#1022=FACE_OUTER_BOUND('',#1563,.T.);
#1023=FACE_OUTER_BOUND('',#1564,.T.);
#1024=FACE_OUTER_BOUND('',#1565,.T.);
#1025=FACE_OUTER_BOUND('',#1566,.T.);
#1026=FACE_OUTER_BOUND('',#1567,.T.);
#1027=FACE_OUTER_BOUND('',#1568,.T.);
#1028=FACE_OUTER_BOUND('',#1569,.T.);
#1029=FACE_OUTER_BOUND('',#1570,.T.);
#1030=FACE_OUTER_BOUND('',#1571,.T.);
#1031=FACE_OUTER_BOUND('',#1572,.T.);
#1032=FACE_OUTER_BOUND('',#1573,.T.);
#1033=FACE_OUTER_BOUND('',#1574,.T.);
#1034=FACE_OUTER_BOUND('',#1575,.T.);
#1035=FACE_OUTER_BOUND('',#1576,.T.);
#1036=FACE_OUTER_BOUND('',#1577,.T.);
#1037=FACE_OUTER_BOUND('',#1578,.T.);
#1038=FACE_OUTER_BOUND('',#1579,.T.);
#1039=FACE_OUTER_BOUND('',#1580,.T.);
#1040=FACE_OUTER_BOUND('',#1581,.T.);
#1041=FACE_OUTER_BOUND('',#1582,.T.);
#1042=FACE_OUTER_BOUND('',#1583,.T.);
#1043=FACE_OUTER_BOUND('',#1584,.T.);
#1044=FACE_OUTER_BOUND('',#1585,.T.);
#1045=FACE_OUTER_BOUND('',#1586,.T.);
#1046=FACE_OUTER_BOUND('',#1587,.T.);
#1047=FACE_OUTER_BOUND('',#1588,.T.);
#1409=EDGE_LOOP('',(#5854,#5855,#5856,#5857));
#1410=EDGE_LOOP('',(#5858,#5859,#5860,#5861));
#1411=EDGE_LOOP('',(#5862,#5863,#5864,#5865));
#1412=EDGE_LOOP('',(#5866,#5867,#5868,#5869));
#1413=EDGE_LOOP('',(#5870,#5871,#5872,#5873));
#1414=EDGE_LOOP('',(#5874,#5875,#5876,#5877));
#1415=EDGE_LOOP('',(#5878,#5879,#5880,#5881));
#1416=EDGE_LOOP('',(#5882,#5883,#5884,#5885));
#1417=EDGE_LOOP('',(#5886,#5887,#5888,#5889));
#1418=EDGE_LOOP('',(#5890,#5891,#5892,#5893));
#1419=EDGE_LOOP('',(#5894,#5895,#5896,#5897));
#1420=EDGE_LOOP('',(#5898,#5899,#5900,#5901));
#1421=EDGE_LOOP('',(#5902,#5903,#5904,#5905,#5906,#5907,#5908,#5909));
#1422=EDGE_LOOP('',(#5910));
#1423=EDGE_LOOP('',(#5911));
#1424=EDGE_LOOP('',(#5912));
#1425=EDGE_LOOP('',(#5913));
#1426=EDGE_LOOP('',(#5914));
#1427=EDGE_LOOP('',(#5915,#5916,#5917,#5918));
#1428=EDGE_LOOP('',(#5919,#5920,#5921,#5922));
#1429=EDGE_LOOP('',(#5923,#5924,#5925,#5926));
#1430=EDGE_LOOP('',(#5927,#5928,#5929,#5930));
#1431=EDGE_LOOP('',(#5931,#5932,#5933,#5934));
#1432=EDGE_LOOP('',(#5935,#5936,#5937,#5938));
#1433=EDGE_LOOP('',(#5939,#5940,#5941,#5942,#5943,#5944,#5945,#5946));
#1434=EDGE_LOOP('',(#5947,#5948,#5949,#5950));
#1435=EDGE_LOOP('',(#5951,#5952,#5953,#5954));
#1436=EDGE_LOOP('',(#5955,#5956,#5957,#5958));
#1437=EDGE_LOOP('',(#5959,#5960,#5961,#5962));
#1438=EDGE_LOOP('',(#5963,#5964,#5965,#5966));
#1439=EDGE_LOOP('',(#5967,#5968,#5969,#5970,#5971,#5972,#5973,#5974,#5975,
#5976,#5977,#5978,#5979));
#1440=EDGE_LOOP('',(#5980,#5981,#5982,#5983,#5984));
#1441=EDGE_LOOP('',(#5985,#5986,#5987,#5988,#5989,#5990,#5991,#5992));
#1442=EDGE_LOOP('',(#5993,#5994,#5995,#5996));
#1443=EDGE_LOOP('',(#5997,#5998,#5999,#6000,#6001,#6002,#6003,#6004));
#1444=EDGE_LOOP('',(#6005,#6006,#6007,#6008));
#1445=EDGE_LOOP('',(#6009,#6010,#6011,#6012,#6013,#6014,#6015));
#1446=EDGE_LOOP('',(#6016,#6017,#6018,#6019));
#1447=EDGE_LOOP('',(#6020,#6021,#6022,#6023,#6024,#6025,#6026,#6027));
#1448=EDGE_LOOP('',(#6028,#6029,#6030,#6031));
#1449=EDGE_LOOP('',(#6032,#6033,#6034,#6035,#6036,#6037));
#1450=EDGE_LOOP('',(#6038,#6039,#6040,#6041));
#1451=EDGE_LOOP('',(#6042,#6043,#6044,#6045,#6046,#6047,#6048,#6049));
#1452=EDGE_LOOP('',(#6050,#6051,#6052,#6053,#6054,#6055));
#1453=EDGE_LOOP('',(#6056,#6057,#6058,#6059,#6060,#6061,#6062,#6063,#6064,
#6065,#6066,#6067,#6068,#6069,#6070,#6071,#6072,#6073,#6074,#6075,#6076,
#6077,#6078,#6079,#6080,#6081,#6082,#6083,#6084,#6085,#6086,#6087,#6088,
#6089));
#1454=EDGE_LOOP('',(#6090,#6091,#6092,#6093,#6094,#6095,#6096,#6097,#6098,
#6099));
#1455=EDGE_LOOP('',(#6100,#6101,#6102,#6103,#6104,#6105,#6106,#6107,#6108,
#6109));
#1456=EDGE_LOOP('',(#6110,#6111,#6112,#6113,#6114,#6115,#6116,#6117,#6118,
#6119,#6120));
#1457=EDGE_LOOP('',(#6121,#6122,#6123,#6124,#6125,#6126,#6127,#6128,#6129,
#6130));
#1458=EDGE_LOOP('',(#6131,#6132,#6133,#6134,#6135,#6136,#6137,#6138,#6139,
#6140,#6141));
#1459=EDGE_LOOP('',(#6142));
#1460=EDGE_LOOP('',(#6143,#6144,#6145,#6146,#6147,#6148,#6149,#6150,#6151,
#6152,#6153));
#1461=EDGE_LOOP('',(#6154,#6155,#6156,#6157,#6158,#6159,#6160,#6161,#6162,
#6163));
#1462=EDGE_LOOP('',(#6164,#6165,#6166,#6167));
#1463=EDGE_LOOP('',(#6168,#6169,#6170,#6171,#6172,#6173,#6174,#6175));
#1464=EDGE_LOOP('',(#6176,#6177,#6178,#6179));
#1465=EDGE_LOOP('',(#6180,#6181,#6182,#6183,#6184,#6185));
#1466=EDGE_LOOP('',(#6186,#6187,#6188,#6189));
#1467=EDGE_LOOP('',(#6190,#6191,#6192,#6193));
#1468=EDGE_LOOP('',(#6194,#6195,#6196,#6197,#6198));
#1469=EDGE_LOOP('',(#6199,#6200,#6201,#6202));
#1470=EDGE_LOOP('',(#6203,#6204,#6205,#6206,#6207,#6208,#6209,#6210));
#1471=EDGE_LOOP('',(#6211,#6212,#6213,#6214));
#1472=EDGE_LOOP('',(#6215,#6216,#6217,#6218));
#1473=EDGE_LOOP('',(#6219,#6220,#6221,#6222));
#1474=EDGE_LOOP('',(#6223,#6224,#6225,#6226));
#1475=EDGE_LOOP('',(#6227,#6228,#6229,#6230));
#1476=EDGE_LOOP('',(#6231,#6232,#6233,#6234));
#1477=EDGE_LOOP('',(#6235,#6236,#6237,#6238));
#1478=EDGE_LOOP('',(#6239,#6240,#6241,#6242,#6243,#6244,#6245,#6246));
#1479=EDGE_LOOP('',(#6247,#6248,#6249,#6250,#6251));
#1480=EDGE_LOOP('',(#6252,#6253,#6254,#6255));
#1481=EDGE_LOOP('',(#6256,#6257,#6258,#6259));
#1482=EDGE_LOOP('',(#6260,#6261,#6262,#6263));
#1483=EDGE_LOOP('',(#6264,#6265,#6266,#6267));
#1484=EDGE_LOOP('',(#6268,#6269,#6270,#6271));
#1485=EDGE_LOOP('',(#6272,#6273,#6274,#6275,#6276));
#1486=EDGE_LOOP('',(#6277,#6278,#6279,#6280,#6281,#6282,#6283,#6284,#6285,
#6286));
#1487=EDGE_LOOP('',(#6287,#6288,#6289,#6290,#6291));
#1488=EDGE_LOOP('',(#6292,#6293,#6294,#6295));
#1489=EDGE_LOOP('',(#6296,#6297,#6298,#6299));
#1490=EDGE_LOOP('',(#6300,#6301,#6302,#6303));
#1491=EDGE_LOOP('',(#6304,#6305,#6306,#6307));
#1492=EDGE_LOOP('',(#6308,#6309,#6310,#6311));
#1493=EDGE_LOOP('',(#6312,#6313,#6314,#6315));
#1494=EDGE_LOOP('',(#6316,#6317,#6318,#6319,#6320,#6321,#6322,#6323,#6324,
#6325));
#1495=EDGE_LOOP('',(#6326,#6327,#6328,#6329,#6330,#6331,#6332));
#1496=EDGE_LOOP('',(#6333,#6334,#6335,#6336));
#1497=EDGE_LOOP('',(#6337,#6338,#6339,#6340));
#1498=EDGE_LOOP('',(#6341,#6342,#6343,#6344));
#1499=EDGE_LOOP('',(#6345,#6346,#6347,#6348));
#1500=EDGE_LOOP('',(#6349,#6350,#6351,#6352));
#1501=EDGE_LOOP('',(#6353,#6354,#6355,#6356));
#1502=EDGE_LOOP('',(#6357,#6358,#6359,#6360));
#1503=EDGE_LOOP('',(#6361,#6362,#6363,#6364));
#1504=EDGE_LOOP('',(#6365,#6366,#6367,#6368));
#1505=EDGE_LOOP('',(#6369,#6370,#6371,#6372));
#1506=EDGE_LOOP('',(#6373,#6374,#6375,#6376));
#1507=EDGE_LOOP('',(#6377,#6378,#6379,#6380));
#1508=EDGE_LOOP('',(#6381,#6382,#6383,#6384));
#1509=EDGE_LOOP('',(#6385,#6386,#6387,#6388));
#1510=EDGE_LOOP('',(#6389,#6390,#6391,#6392));
#1511=EDGE_LOOP('',(#6393,#6394,#6395,#6396,#6397,#6398,#6399,#6400,#6401,
#6402));
#1512=EDGE_LOOP('',(#6403,#6404,#6405,#6406));
#1513=EDGE_LOOP('',(#6407,#6408,#6409,#6410));
#1514=EDGE_LOOP('',(#6411,#6412,#6413,#6414));
#1515=EDGE_LOOP('',(#6415,#6416,#6417,#6418));
#1516=EDGE_LOOP('',(#6419,#6420,#6421,#6422));
#1517=EDGE_LOOP('',(#6423,#6424,#6425,#6426));
#1518=EDGE_LOOP('',(#6427,#6428,#6429,#6430));
#1519=EDGE_LOOP('',(#6431,#6432,#6433,#6434));
#1520=EDGE_LOOP('',(#6435,#6436,#6437,#6438));
#1521=EDGE_LOOP('',(#6439,#6440,#6441,#6442));
#1522=EDGE_LOOP('',(#6443,#6444,#6445,#6446,#6447,#6448,#6449,#6450,#6451,
#6452));
#1523=EDGE_LOOP('',(#6453,#6454,#6455,#6456));
#1524=EDGE_LOOP('',(#6457,#6458,#6459,#6460));
#1525=EDGE_LOOP('',(#6461,#6462,#6463,#6464));
#1526=EDGE_LOOP('',(#6465,#6466,#6467,#6468));
#1527=EDGE_LOOP('',(#6469,#6470,#6471,#6472));
#1528=EDGE_LOOP('',(#6473,#6474,#6475,#6476));
#1529=EDGE_LOOP('',(#6477,#6478,#6479,#6480));
#1530=EDGE_LOOP('',(#6481,#6482,#6483,#6484));
#1531=EDGE_LOOP('',(#6485,#6486,#6487,#6488));
#1532=EDGE_LOOP('',(#6489,#6490,#6491,#6492));
#1533=EDGE_LOOP('',(#6493,#6494,#6495,#6496));
#1534=EDGE_LOOP('',(#6497,#6498,#6499,#6500,#6501,#6502,#6503,#6504,#6505,
#6506,#6507));
#1535=EDGE_LOOP('',(#6508,#6509,#6510,#6511));
#1536=EDGE_LOOP('',(#6512,#6513,#6514,#6515));
#1537=EDGE_LOOP('',(#6516,#6517,#6518,#6519));
#1538=EDGE_LOOP('',(#6520,#6521,#6522,#6523));
#1539=EDGE_LOOP('',(#6524,#6525,#6526,#6527));
#1540=EDGE_LOOP('',(#6528,#6529,#6530,#6531));
#1541=EDGE_LOOP('',(#6532,#6533,#6534,#6535));
#1542=EDGE_LOOP('',(#6536,#6537,#6538,#6539));
#1543=EDGE_LOOP('',(#6540,#6541,#6542,#6543));
#1544=EDGE_LOOP('',(#6544,#6545,#6546,#6547));
#1545=EDGE_LOOP('',(#6548,#6549,#6550,#6551,#6552,#6553,#6554,#6555,#6556,
#6557));
#1546=EDGE_LOOP('',(#6558,#6559,#6560,#6561));
#1547=EDGE_LOOP('',(#6562,#6563,#6564,#6565));
#1548=EDGE_LOOP('',(#6566,#6567,#6568,#6569));
#1549=EDGE_LOOP('',(#6570,#6571,#6572,#6573));
#1550=EDGE_LOOP('',(#6574,#6575,#6576,#6577));
#1551=EDGE_LOOP('',(#6578,#6579,#6580,#6581));
#1552=EDGE_LOOP('',(#6582,#6583,#6584,#6585));
#1553=EDGE_LOOP('',(#6586,#6587,#6588,#6589));
#1554=EDGE_LOOP('',(#6590,#6591,#6592,#6593));
#1555=EDGE_LOOP('',(#6594,#6595,#6596,#6597));
#1556=EDGE_LOOP('',(#6598,#6599,#6600,#6601));
#1557=EDGE_LOOP('',(#6602,#6603,#6604,#6605,#6606,#6607,#6608,#6609,#6610,
#6611,#6612));
#1558=EDGE_LOOP('',(#6613,#6614,#6615,#6616));
#1559=EDGE_LOOP('',(#6617,#6618,#6619,#6620));
#1560=EDGE_LOOP('',(#6621,#6622,#6623,#6624));
#1561=EDGE_LOOP('',(#6625,#6626,#6627,#6628));
#1562=EDGE_LOOP('',(#6629,#6630,#6631,#6632));
#1563=EDGE_LOOP('',(#6633,#6634,#6635,#6636));
#1564=EDGE_LOOP('',(#6637,#6638,#6639,#6640));
#1565=EDGE_LOOP('',(#6641,#6642,#6643,#6644));
#1566=EDGE_LOOP('',(#6645,#6646,#6647,#6648));
#1567=EDGE_LOOP('',(#6649,#6650,#6651,#6652));
#1568=EDGE_LOOP('',(#6653,#6654,#6655,#6656,#6657,#6658,#6659,#6660,#6661,
#6662));
#1569=EDGE_LOOP('',(#6663,#6664,#6665,#6666));
#1570=EDGE_LOOP('',(#6667,#6668,#6669,#6670));
#1571=EDGE_LOOP('',(#6671,#6672,#6673,#6674));
#1572=EDGE_LOOP('',(#6675,#6676,#6677,#6678));
#1573=EDGE_LOOP('',(#6679,#6680,#6681,#6682));
#1574=EDGE_LOOP('',(#6683,#6684,#6685,#6686));
#1575=EDGE_LOOP('',(#6687,#6688,#6689,#6690));
#1576=EDGE_LOOP('',(#6691,#6692,#6693,#6694));
#1577=EDGE_LOOP('',(#6695,#6696,#6697,#6698));
#1578=EDGE_LOOP('',(#6699,#6700,#6701,#6702));
#1579=EDGE_LOOP('',(#6703,#6704,#6705,#6706));
#1580=EDGE_LOOP('',(#6707,#6708,#6709,#6710,#6711,#6712,#6713,#6714,#6715,
#6716,#6717));
#1581=EDGE_LOOP('',(#6718,#6719,#6720,#6721));
#1582=EDGE_LOOP('',(#6722,#6723,#6724,#6725));
#1583=EDGE_LOOP('',(#6726,#6727,#6728,#6729));
#1584=EDGE_LOOP('',(#6730,#6731,#6732,#6733));
#1585=EDGE_LOOP('',(#6734,#6735,#6736,#6737));
#1586=EDGE_LOOP('',(#6738,#6739,#6740,#6741));
#1587=EDGE_LOOP('',(#6742,#6743,#6744,#6745));
#1588=EDGE_LOOP('',(#6746,#6747,#6748,#6749));
#1999=LINE('',#12444,#2844);
#2000=LINE('',#12446,#2845);
#2001=LINE('',#12448,#2846);
#2002=LINE('',#12449,#2847);
#2003=LINE('',#12454,#2848);
#2004=LINE('',#12459,#2849);
#2005=LINE('',#12460,#2850);
#2006=LINE('',#12461,#2851);
#2007=LINE('',#12466,#2852);
#2008=LINE('',#12471,#2853);
#2009=LINE('',#12472,#2854);
#2010=LINE('',#12473,#2855);
#2011=LINE('',#12478,#2856);
#2012=LINE('',#12483,#2857);
#2013=LINE('',#12484,#2858);
#2014=LINE('',#12485,#2859);
#2015=LINE('',#12491,#2860);
#2016=LINE('',#12494,#2861);
#2017=LINE('',#12497,#2862);
#2018=LINE('',#12498,#2863);
#2019=LINE('',#12501,#2864);
#2020=LINE('',#12505,#2865);
#2021=LINE('',#12506,#2866);
#2022=LINE('',#12520,#2867);
#2023=LINE('',#12522,#2868);
#2024=LINE('',#12524,#2869);
#2025=LINE('',#12525,#2870);
#2026=LINE('',#12528,#2871);
#2027=LINE('',#12532,#2872);
#2028=LINE('',#12533,#2873);
#2029=LINE('',#12536,#2874);
#2030=LINE('',#12540,#2875);
#2031=LINE('',#12541,#2876);
#2032=LINE('',#12545,#2877);
#2033=LINE('',#12555,#2878);
#2034=LINE('',#12557,#2879);
#2035=LINE('',#12559,#2880);
#2036=LINE('',#12561,#2881);
#2037=LINE('',#12567,#2882);
#2038=LINE('',#12572,#2883);
#2039=LINE('',#12575,#2884);
#2040=LINE('',#12578,#2885);
#2041=LINE('',#12581,#2886);
#2042=LINE('',#12582,#2887);
#2043=LINE('',#12585,#2888);
#2044=LINE('',#12589,#2889);
#2045=LINE('',#12591,#2890);
#2046=LINE('',#12593,#2891);
#2047=LINE('',#12595,#2892);
#2048=LINE('',#12597,#2893);
#2049=LINE('',#12599,#2894);
#2050=LINE('',#12601,#2895);
#2051=LINE('',#12603,#2896);
#2052=LINE('',#12605,#2897);
#2053=LINE('',#12607,#2898);
#2054=LINE('',#12637,#2899);
#2055=LINE('',#12662,#2900);
#2056=LINE('',#12686,#2901);
#2057=LINE('',#12691,#2902);
#2058=LINE('',#12715,#2903);
#2059=LINE('',#12718,#2904);
#2060=LINE('',#12721,#2905);
#2061=LINE('',#12723,#2906);
#2062=LINE('',#12725,#2907);
#2063=LINE('',#12726,#2908);
#2064=LINE('',#12729,#2909);
#2065=LINE('',#12735,#2910);
#2066=LINE('',#12759,#2911);
#2067=LINE('',#12760,#2912);
#2068=LINE('',#12763,#2913);
#2069=LINE('',#12768,#2914);
#2070=LINE('',#12771,#2915);
#2071=LINE('',#12777,#2916);
#2072=LINE('',#12804,#2917);
#2073=LINE('',#12805,#2918);
#2074=LINE('',#12806,#2919);
#2075=LINE('',#12809,#2920);
#2076=LINE('',#12811,#2921);
#2077=LINE('',#12836,#2922);
#2078=LINE('',#12838,#2923);
#2079=LINE('',#12840,#2924);
#2080=LINE('',#12842,#2925);
#2081=LINE('',#12844,#2926);
#2082=LINE('',#12846,#2927);
#2083=LINE('',#12848,#2928);
#2084=LINE('',#12850,#2929);
#2085=LINE('',#12852,#2930);
#2086=LINE('',#12854,#2931);
#2087=LINE('',#12856,#2932);
#2088=LINE('',#12858,#2933);
#2089=LINE('',#12860,#2934);
#2090=LINE('',#12862,#2935);
#2091=LINE('',#12863,#2936);
#2092=LINE('',#12866,#2937);
#2093=LINE('',#12868,#2938);
#2094=LINE('',#12870,#2939);
#2095=LINE('',#12872,#2940);
#2096=LINE('',#12874,#2941);
#2097=LINE('',#12876,#2942);
#2098=LINE('',#12878,#2943);
#2099=LINE('',#12880,#2944);
#2100=LINE('',#12882,#2945);
#2101=LINE('',#12883,#2946);
#2102=LINE('',#12886,#2947);
#2103=LINE('',#12888,#2948);
#2104=LINE('',#12890,#2949);
#2105=LINE('',#12892,#2950);
#2106=LINE('',#12894,#2951);
#2107=LINE('',#12896,#2952);
#2108=LINE('',#12898,#2953);
#2109=LINE('',#12900,#2954);
#2110=LINE('',#12902,#2955);
#2111=LINE('',#12903,#2956);
#2112=LINE('',#12950,#2957);
#2113=LINE('',#12952,#2958);
#2114=LINE('',#12954,#2959);
#2115=LINE('',#12956,#2960);
#2116=LINE('',#12958,#2961);
#2117=LINE('',#12960,#2962);
#2118=LINE('',#12962,#2963);
#2119=LINE('',#12964,#2964);
#2120=LINE('',#12966,#2965);
#2121=LINE('',#12967,#2966);
#2122=LINE('',#13060,#2967);
#2123=LINE('',#13062,#2968);
#2124=LINE('',#13064,#2969);
#2125=LINE('',#13066,#2970);
#2126=LINE('',#13068,#2971);
#2127=LINE('',#13070,#2972);
#2128=LINE('',#13072,#2973);
#2129=LINE('',#13074,#2974);
#2130=LINE('',#13076,#2975);
#2131=LINE('',#13077,#2976);
#2132=LINE('',#13080,#2977);
#2133=LINE('',#13086,#2978);
#2134=LINE('',#13106,#2979);
#2135=LINE('',#13109,#2980);
#2136=LINE('',#13111,#2981);
#2137=LINE('',#13113,#2982);
#2138=LINE('',#13114,#2983);
#2139=LINE('',#13117,#2984);
#2140=LINE('',#13118,#2985);
#2141=LINE('',#13121,#2986);
#2142=LINE('',#13122,#2987);
#2143=LINE('',#13125,#2988);
#2144=LINE('',#13128,#2989);
#2145=LINE('',#13129,#2990);
#2146=LINE('',#13133,#2991);
#2147=LINE('',#13135,#2992);
#2148=LINE('',#13137,#2993);
#2149=LINE('',#13141,#2994);
#2150=LINE('',#13142,#2995);
#2151=LINE('',#13145,#2996);
#2152=LINE('',#13146,#2997);
#2153=LINE('',#13173,#2998);
#2154=LINE('',#13174,#2999);
#2155=LINE('',#13177,#3000);
#2156=LINE('',#13178,#3001);
#2157=LINE('',#13181,#3002);
#2158=LINE('',#13182,#3003);
#2159=LINE('',#13185,#3004);
#2160=LINE('',#13186,#3005);
#2161=LINE('',#13189,#3006);
#2162=LINE('',#13190,#3007);
#2163=LINE('',#13193,#3008);
#2164=LINE('',#13194,#3009);
#2165=LINE('',#13196,#3010);
#2166=LINE('',#13200,#3011);
#2167=LINE('',#13201,#3012);
#2168=LINE('',#13204,#3013);
#2169=LINE('',#13205,#3014);
#2170=LINE('',#13208,#3015);
#2171=LINE('',#13209,#3016);
#2172=LINE('',#13212,#3017);
#2173=LINE('',#13213,#3018);
#2174=LINE('',#13216,#3019);
#2175=LINE('',#13217,#3020);
#2176=LINE('',#13220,#3021);
#2177=LINE('',#13221,#3022);
#2178=LINE('',#13223,#3023);
#2179=LINE('',#13239,#3024);
#2180=LINE('',#13246,#3025);
#2181=LINE('',#13253,#3026);
#2182=LINE('',#13260,#3027);
#2183=LINE('',#13267,#3028);
#2184=LINE('',#13276,#3029);
#2185=LINE('',#13278,#3030);
#2186=LINE('',#13279,#3031);
#2187=LINE('',#13282,#3032);
#2188=LINE('',#13283,#3033);
#2189=LINE('',#13286,#3034);
#2190=LINE('',#13287,#3035);
#2191=LINE('',#13290,#3036);
#2192=LINE('',#13291,#3037);
#2193=LINE('',#13294,#3038);
#2194=LINE('',#13295,#3039);
#2195=LINE('',#13298,#3040);
#2196=LINE('',#13299,#3041);
#2197=LINE('',#13302,#3042);
#2198=LINE('',#13303,#3043);
#2199=LINE('',#13306,#3044);
#2200=LINE('',#13307,#3045);
#2201=LINE('',#13310,#3046);
#2202=LINE('',#13311,#3047);
#2203=LINE('',#13313,#3048);
#2204=LINE('',#13317,#3049);
#2205=LINE('',#13319,#3050);
#2206=LINE('',#13320,#3051);
#2207=LINE('',#13323,#3052);
#2208=LINE('',#13324,#3053);
#2209=LINE('',#13327,#3054);
#2210=LINE('',#13328,#3055);
#2211=LINE('',#13331,#3056);
#2212=LINE('',#13332,#3057);
#2213=LINE('',#13335,#3058);
#2214=LINE('',#13336,#3059);
#2215=LINE('',#13339,#3060);
#2216=LINE('',#13340,#3061);
#2217=LINE('',#13343,#3062);
#2218=LINE('',#13344,#3063);
#2219=LINE('',#13347,#3064);
#2220=LINE('',#13348,#3065);
#2221=LINE('',#13351,#3066);
#2222=LINE('',#13352,#3067);
#2223=LINE('',#13354,#3068);
#2224=LINE('',#13363,#3069);
#2225=LINE('',#13368,#3070);
#2226=LINE('',#13376,#3071);
#2227=LINE('',#13387,#3072);
#2228=LINE('',#13398,#3073);
#2229=LINE('',#13409,#3074);
#2230=LINE('',#13420,#3075);
#2231=LINE('',#13431,#3076);
#2232=LINE('',#13442,#3077);
#2233=LINE('',#13453,#3078);
#2234=LINE('',#13464,#3079);
#2235=LINE('',#13480,#3080);
#2236=LINE('',#13482,#3081);
#2237=LINE('',#13483,#3082);
#2238=LINE('',#13486,#3083);
#2239=LINE('',#13487,#3084);
#2240=LINE('',#13490,#3085);
#2241=LINE('',#13491,#3086);
#2242=LINE('',#13494,#3087);
#2243=LINE('',#13495,#3088);
#2244=LINE('',#13498,#3089);
#2245=LINE('',#13499,#3090);
#2246=LINE('',#13502,#3091);
#2247=LINE('',#13503,#3092);
#2248=LINE('',#13506,#3093);
#2249=LINE('',#13507,#3094);
#2250=LINE('',#13510,#3095);
#2251=LINE('',#13511,#3096);
#2252=LINE('',#13514,#3097);
#2253=LINE('',#13515,#3098);
#2254=LINE('',#13517,#3099);
#2255=LINE('',#13526,#3100);
#2256=LINE('',#13531,#3101);
#2257=LINE('',#13539,#3102);
#2258=LINE('',#13550,#3103);
#2259=LINE('',#13561,#3104);
#2260=LINE('',#13572,#3105);
#2261=LINE('',#13583,#3106);
#2262=LINE('',#13594,#3107);
#2263=LINE('',#13605,#3108);
#2264=LINE('',#13616,#3109);
#2265=LINE('',#13627,#3110);
#2266=LINE('',#13643,#3111);
#2267=LINE('',#13645,#3112);
#2268=LINE('',#13646,#3113);
#2269=LINE('',#13649,#3114);
#2270=LINE('',#13650,#3115);
#2271=LINE('',#13653,#3116);
#2272=LINE('',#13654,#3117);
#2273=LINE('',#13657,#3118);
#2274=LINE('',#13658,#3119);
#2275=LINE('',#13661,#3120);
#2276=LINE('',#13662,#3121);
#2277=LINE('',#13665,#3122);
#2278=LINE('',#13666,#3123);
#2279=LINE('',#13669,#3124);
#2280=LINE('',#13670,#3125);
#2281=LINE('',#13673,#3126);
#2282=LINE('',#13674,#3127);
#2283=LINE('',#13677,#3128);
#2284=LINE('',#13678,#3129);
#2285=LINE('',#13680,#3130);
#2286=LINE('',#13689,#3131);
#2287=LINE('',#13694,#3132);
#2288=LINE('',#13702,#3133);
#2289=LINE('',#13713,#3134);
#2290=LINE('',#13724,#3135);
#2291=LINE('',#13735,#3136);
#2292=LINE('',#13746,#3137);
#2293=LINE('',#13757,#3138);
#2294=LINE('',#13768,#3139);
#2295=LINE('',#13779,#3140);
#2296=LINE('',#13790,#3141);
#2297=LINE('',#13805,#3142);
#2298=LINE('',#13807,#3143);
#2299=LINE('',#13809,#3144);
#2300=LINE('',#13811,#3145);
#2301=LINE('',#13813,#3146);
#2302=LINE('',#13815,#3147);
#2303=LINE('',#13817,#3148);
#2844=VECTOR('',#10157,10.);
#2845=VECTOR('',#10158,10.);
#2846=VECTOR('',#10159,10.);
#2847=VECTOR('',#10160,10.);
#2848=VECTOR('',#10165,10.);
#2849=VECTOR('',#10170,10.);
#2850=VECTOR('',#10171,10.);
#2851=VECTOR('',#10172,10.);
#2852=VECTOR('',#10177,10.);
#2853=VECTOR('',#10182,10.);
#2854=VECTOR('',#10183,10.);
#2855=VECTOR('',#10184,10.);
#2856=VECTOR('',#10189,10.);
#2857=VECTOR('',#10194,10.);
#2858=VECTOR('',#10195,10.);
#2859=VECTOR('',#10196,10.);
#2860=VECTOR('',#10205,10.);
#2861=VECTOR('',#10208,10.);
#2862=VECTOR('',#10211,10.);
#2863=VECTOR('',#10212,10.);
#2864=VECTOR('',#10215,10.);
#2865=VECTOR('',#10220,10.);
#2866=VECTOR('',#10221,10.);
#2867=VECTOR('',#10236,10.);
#2868=VECTOR('',#10237,10.);
#2869=VECTOR('',#10238,10.);
#2870=VECTOR('',#10239,10.);
#2871=VECTOR('',#10242,10.);
#2872=VECTOR('',#10247,10.);
#2873=VECTOR('',#10248,10.);
#2874=VECTOR('',#10251,10.);
#2875=VECTOR('',#10256,10.);
#2876=VECTOR('',#10257,10.);
#2877=VECTOR('',#10260,10.);
#2878=VECTOR('',#10267,10.);
#2879=VECTOR('',#10268,10.);
#2880=VECTOR('',#10269,10.);
#2881=VECTOR('',#10270,10.);
#2882=VECTOR('',#10271,10.);
#2883=VECTOR('',#10280,10.);
#2884=VECTOR('',#10283,10.);
#2885=VECTOR('',#10286,10.);
#2886=VECTOR('',#10289,10.);
#2887=VECTOR('',#10290,10.);
#2888=VECTOR('',#10293,10.);
#2889=VECTOR('',#10298,10.);
#2890=VECTOR('',#10299,10.);
#2891=VECTOR('',#10300,10.);
#2892=VECTOR('',#10301,10.);
#2893=VECTOR('',#10302,10.);
#2894=VECTOR('',#10303,10.);
#2895=VECTOR('',#10304,10.);
#2896=VECTOR('',#10305,10.);
#2897=VECTOR('',#10306,10.);
#2898=VECTOR('',#10307,10.);
#2899=VECTOR('',#10310,10.);
#2900=VECTOR('',#10311,10.);
#2901=VECTOR('',#10314,10.);
#2902=VECTOR('',#10319,3.27928932188134);
#2903=VECTOR('',#10326,10.);
#2904=VECTOR('',#10329,10.);
#2905=VECTOR('',#10332,10.);
#2906=VECTOR('',#10333,10.);
#2907=VECTOR('',#10334,10.);
#2908=VECTOR('',#10335,10.);
#2909=VECTOR('',#10338,2.475);
#2910=VECTOR('',#10345,3.27928932188134);
#2911=VECTOR('',#10352,10.);
#2912=VECTOR('',#10353,10.);
#2913=VECTOR('',#10356,10.);
#2914=VECTOR('',#10357,10.);
#2915=VECTOR('',#10360,2.475);
#2916=VECTOR('',#10367,3.27928932188134);
#2917=VECTOR('',#10372,10.);
#2918=VECTOR('',#10373,10.);
#2919=VECTOR('',#10374,10.);
#2920=VECTOR('',#10377,10.);
#2921=VECTOR('',#10380,10.);
#2922=VECTOR('',#10381,10.);
#2923=VECTOR('',#10382,10.);
#2924=VECTOR('',#10383,10.);
#2925=VECTOR('',#10384,10.);
#2926=VECTOR('',#10385,10.);
#2927=VECTOR('',#10386,10.);
#2928=VECTOR('',#10387,10.);
#2929=VECTOR('',#10388,10.);
#2930=VECTOR('',#10389,10.);
#2931=VECTOR('',#10390,10.);
#2932=VECTOR('',#10391,10.);
#2933=VECTOR('',#10392,10.);
#2934=VECTOR('',#10393,10.);
#2935=VECTOR('',#10394,10.);
#2936=VECTOR('',#10395,10.);
#2937=VECTOR('',#10396,10.);
#2938=VECTOR('',#10397,10.);
#2939=VECTOR('',#10398,10.);
#2940=VECTOR('',#10399,10.);
#2941=VECTOR('',#10400,10.);
#2942=VECTOR('',#10401,10.);
#2943=VECTOR('',#10402,10.);
#2944=VECTOR('',#10403,10.);
#2945=VECTOR('',#10404,10.);
#2946=VECTOR('',#10405,10.);
#2947=VECTOR('',#10406,10.);
#2948=VECTOR('',#10407,10.);
#2949=VECTOR('',#10408,10.);
#2950=VECTOR('',#10409,10.);
#2951=VECTOR('',#10410,10.);
#2952=VECTOR('',#10411,10.);
#2953=VECTOR('',#10412,10.);
#2954=VECTOR('',#10413,10.);
#2955=VECTOR('',#10414,10.);
#2956=VECTOR('',#10415,10.);
#2957=VECTOR('',#10416,10.);
#2958=VECTOR('',#10417,10.);
#2959=VECTOR('',#10418,10.);
#2960=VECTOR('',#10419,10.);
#2961=VECTOR('',#10420,10.);
#2962=VECTOR('',#10421,10.);
#2963=VECTOR('',#10422,10.);
#2964=VECTOR('',#10423,10.);
#2965=VECTOR('',#10424,10.);
#2966=VECTOR('',#10425,10.);
#2967=VECTOR('',#10428,10.);
#2968=VECTOR('',#10429,10.);
#2969=VECTOR('',#10430,10.);
#2970=VECTOR('',#10431,10.);
#2971=VECTOR('',#10432,10.);
#2972=VECTOR('',#10433,10.);
#2973=VECTOR('',#10434,10.);
#2974=VECTOR('',#10435,10.);
#2975=VECTOR('',#10436,10.);
#2976=VECTOR('',#10437,10.);
#2977=VECTOR('',#10440,2.475);
#2978=VECTOR('',#10447,3.27928932188134);
#2979=VECTOR('',#10450,2.475);
#2980=VECTOR('',#10455,10.);
#2981=VECTOR('',#10456,10.);
#2982=VECTOR('',#10457,10.);
#2983=VECTOR('',#10458,10.);
#2984=VECTOR('',#10461,10.);
#2985=VECTOR('',#10462,10.);
#2986=VECTOR('',#10465,10.);
#2987=VECTOR('',#10466,10.);
#2988=VECTOR('',#10471,10.);
#2989=VECTOR('',#10474,10.);
#2990=VECTOR('',#10475,10.);
#2991=VECTOR('',#10482,10.);
#2992=VECTOR('',#10485,10.);
#2993=VECTOR('',#10488,10.);
#2994=VECTOR('',#10493,10.);
#2995=VECTOR('',#10494,10.);
#2996=VECTOR('',#10497,10.);
#2997=VECTOR('',#10498,10.);
#2998=VECTOR('',#10503,10.);
#2999=VECTOR('',#10504,10.);
#3000=VECTOR('',#10507,10.);
#3001=VECTOR('',#10508,10.);
#3002=VECTOR('',#10511,10.);
#3003=VECTOR('',#10512,10.);
#3004=VECTOR('',#10515,10.);
#3005=VECTOR('',#10516,10.);
#3006=VECTOR('',#10519,10.);
#3007=VECTOR('',#10520,10.);
#3008=VECTOR('',#10523,10.);
#3009=VECTOR('',#10524,10.);
#3010=VECTOR('',#10527,10.);
#3011=VECTOR('',#10532,10.);
#3012=VECTOR('',#10533,10.);
#3013=VECTOR('',#10536,10.);
#3014=VECTOR('',#10537,10.);
#3015=VECTOR('',#10540,10.);
#3016=VECTOR('',#10541,10.);
#3017=VECTOR('',#10544,10.);
#3018=VECTOR('',#10545,10.);
#3019=VECTOR('',#10548,10.);
#3020=VECTOR('',#10549,10.);
#3021=VECTOR('',#10552,10.);
#3022=VECTOR('',#10553,10.);
#3023=VECTOR('',#10556,10.);
#3024=VECTOR('',#10559,10.);
#3025=VECTOR('',#10560,10.);
#3026=VECTOR('',#10561,10.);
#3027=VECTOR('',#10562,10.);
#3028=VECTOR('',#10563,10.);
#3029=VECTOR('',#10566,10.);
#3030=VECTOR('',#10567,10.);
#3031=VECTOR('',#10568,10.);
#3032=VECTOR('',#10571,10.);
#3033=VECTOR('',#10572,10.);
#3034=VECTOR('',#10575,10.);
#3035=VECTOR('',#10576,10.);
#3036=VECTOR('',#10579,10.);
#3037=VECTOR('',#10580,10.);
#3038=VECTOR('',#10583,10.);
#3039=VECTOR('',#10584,10.);
#3040=VECTOR('',#10587,10.);
#3041=VECTOR('',#10588,10.);
#3042=VECTOR('',#10591,10.);
#3043=VECTOR('',#10592,10.);
#3044=VECTOR('',#10595,10.);
#3045=VECTOR('',#10596,10.);
#3046=VECTOR('',#10599,10.);
#3047=VECTOR('',#10600,10.);
#3048=VECTOR('',#10603,10.);
#3049=VECTOR('',#10608,10.);
#3050=VECTOR('',#10609,10.);
#3051=VECTOR('',#10610,10.);
#3052=VECTOR('',#10613,10.);
#3053=VECTOR('',#10614,10.);
#3054=VECTOR('',#10617,10.);
#3055=VECTOR('',#10618,10.);
#3056=VECTOR('',#10621,10.);
#3057=VECTOR('',#10622,10.);
#3058=VECTOR('',#10625,10.);
#3059=VECTOR('',#10626,10.);
#3060=VECTOR('',#10629,10.);
#3061=VECTOR('',#10630,10.);
#3062=VECTOR('',#10633,10.);
#3063=VECTOR('',#10634,10.);
#3064=VECTOR('',#10637,10.);
#3065=VECTOR('',#10638,10.);
#3066=VECTOR('',#10641,10.);
#3067=VECTOR('',#10642,10.);
#3068=VECTOR('',#10645,10.);
#3069=VECTOR('',#10648,10.);
#3070=VECTOR('',#10649,10.);
#3071=VECTOR('',#10650,10.);
#3072=VECTOR('',#10651,10.);
#3073=VECTOR('',#10652,10.);
#3074=VECTOR('',#10653,10.);
#3075=VECTOR('',#10654,10.);
#3076=VECTOR('',#10655,10.);
#3077=VECTOR('',#10656,10.);
#3078=VECTOR('',#10657,10.);
#3079=VECTOR('',#10658,10.);
#3080=VECTOR('',#10663,10.);
#3081=VECTOR('',#10664,10.);
#3082=VECTOR('',#10665,10.);
#3083=VECTOR('',#10668,10.);
#3084=VECTOR('',#10669,10.);
#3085=VECTOR('',#10672,10.);
#3086=VECTOR('',#10673,10.);
#3087=VECTOR('',#10676,10.);
#3088=VECTOR('',#10677,10.);
#3089=VECTOR('',#10680,10.);
#3090=VECTOR('',#10681,10.);
#3091=VECTOR('',#10684,10.);
#3092=VECTOR('',#10685,10.);
#3093=VECTOR('',#10688,10.);
#3094=VECTOR('',#10689,10.);
#3095=VECTOR('',#10692,10.);
#3096=VECTOR('',#10693,10.);
#3097=VECTOR('',#10696,10.);
#3098=VECTOR('',#10697,10.);
#3099=VECTOR('',#10700,10.);
#3100=VECTOR('',#10703,10.);
#3101=VECTOR('',#10704,10.);
#3102=VECTOR('',#10705,10.);
#3103=VECTOR('',#10706,10.);
#3104=VECTOR('',#10707,10.);
#3105=VECTOR('',#10708,10.);
#3106=VECTOR('',#10709,10.);
#3107=VECTOR('',#10710,10.);
#3108=VECTOR('',#10711,10.);
#3109=VECTOR('',#10712,10.);
#3110=VECTOR('',#10713,10.);
#3111=VECTOR('',#10718,10.);
#3112=VECTOR('',#10719,10.);
#3113=VECTOR('',#10720,10.);
#3114=VECTOR('',#10723,10.);
#3115=VECTOR('',#10724,10.);
#3116=VECTOR('',#10727,10.);
#3117=VECTOR('',#10728,10.);
#3118=VECTOR('',#10731,10.);
#3119=VECTOR('',#10732,10.);
#3120=VECTOR('',#10735,10.);
#3121=VECTOR('',#10736,10.);
#3122=VECTOR('',#10739,10.);
#3123=VECTOR('',#10740,10.);
#3124=VECTOR('',#10743,10.);
#3125=VECTOR('',#10744,10.);
#3126=VECTOR('',#10747,10.);
#3127=VECTOR('',#10748,10.);
#3128=VECTOR('',#10751,10.);
#3129=VECTOR('',#10752,10.);
#3130=VECTOR('',#10755,10.);
#3131=VECTOR('',#10758,10.);
#3132=VECTOR('',#10759,10.);
#3133=VECTOR('',#10760,10.);
#3134=VECTOR('',#10761,10.);
#3135=VECTOR('',#10762,10.);
#3136=VECTOR('',#10763,10.);
#3137=VECTOR('',#10764,10.);
#3138=VECTOR('',#10765,10.);
#3139=VECTOR('',#10766,10.);
#3140=VECTOR('',#10767,10.);
#3141=VECTOR('',#10768,10.);
#3142=VECTOR('',#10773,1.7);
#3143=VECTOR('',#10776,1.7);
#3144=VECTOR('',#10779,1.7);
#3145=VECTOR('',#10782,1.7);
#3146=VECTOR('',#10785,6.5);
#3147=VECTOR('',#10788,10.);
#3148=VECTOR('',#10791,10.);
#3672=VERTEX_POINT('',#12442);
#3673=VERTEX_POINT('',#12443);
#3674=VERTEX_POINT('',#12445);
#3675=VERTEX_POINT('',#12447);
#3676=VERTEX_POINT('',#12451);
#3677=VERTEX_POINT('',#12453);
#3678=VERTEX_POINT('',#12457);
#3679=VERTEX_POINT('',#12458);
#3680=VERTEX_POINT('',#12463);
#3681=VERTEX_POINT('',#12465);
#3682=VERTEX_POINT('',#12469);
#3683=VERTEX_POINT('',#12470);
#3684=VERTEX_POINT('',#12475);
#3685=VERTEX_POINT('',#12477);
#3686=VERTEX_POINT('',#12481);
#3687=VERTEX_POINT('',#12482);
#3688=VERTEX_POINT('',#12490);
#3689=VERTEX_POINT('',#12492);
#3690=VERTEX_POINT('',#12496);
#3691=VERTEX_POINT('',#12500);
#3692=VERTEX_POINT('',#12504);
#3693=VERTEX_POINT('',#12508);
#3694=VERTEX_POINT('',#12510);
#3695=VERTEX_POINT('',#12512);
#3696=VERTEX_POINT('',#12514);
#3697=VERTEX_POINT('',#12516);
#3698=VERTEX_POINT('',#12519);
#3699=VERTEX_POINT('',#12521);
#3700=VERTEX_POINT('',#12523);
#3701=VERTEX_POINT('',#12527);
#3702=VERTEX_POINT('',#12531);
#3703=VERTEX_POINT('',#12535);
#3704=VERTEX_POINT('',#12539);
#3705=VERTEX_POINT('',#12543);
#3706=VERTEX_POINT('',#12544);
#3707=VERTEX_POINT('',#12549);
#3708=VERTEX_POINT('',#12550);
#3709=VERTEX_POINT('',#12556);
#3710=VERTEX_POINT('',#12558);
#3711=VERTEX_POINT('',#12560);
#3712=VERTEX_POINT('',#12562);
#3713=VERTEX_POINT('',#12574);
#3714=VERTEX_POINT('',#12576);
#3715=VERTEX_POINT('',#12580);
#3716=VERTEX_POINT('',#12584);
#3717=VERTEX_POINT('',#12588);
#3718=VERTEX_POINT('',#12590);
#3719=VERTEX_POINT('',#12592);
#3720=VERTEX_POINT('',#12594);
#3721=VERTEX_POINT('',#12596);
#3722=VERTEX_POINT('',#12598);
#3723=VERTEX_POINT('',#12600);
#3724=VERTEX_POINT('',#12602);
#3725=VERTEX_POINT('',#12604);
#3726=VERTEX_POINT('',#12606);
#3727=VERTEX_POINT('',#12608);
#3728=VERTEX_POINT('',#12624);
#3729=VERTEX_POINT('',#12632);
#3730=VERTEX_POINT('',#12652);
#3731=VERTEX_POINT('',#12657);
#3732=VERTEX_POINT('',#12661);
#3733=VERTEX_POINT('',#12663);
#3734=VERTEX_POINT('',#12675);
#3735=VERTEX_POINT('',#12688);
#3736=VERTEX_POINT('',#12690);
#3737=VERTEX_POINT('',#12692);
#3738=VERTEX_POINT('',#12694);
#3739=VERTEX_POINT('',#12698);
#3740=VERTEX_POINT('',#12709);
#3741=VERTEX_POINT('',#12716);
#3742=VERTEX_POINT('',#12720);
#3743=VERTEX_POINT('',#12722);
#3744=VERTEX_POINT('',#12724);
#3745=VERTEX_POINT('',#12728);
#3746=VERTEX_POINT('',#12732);
#3747=VERTEX_POINT('',#12734);
#3748=VERTEX_POINT('',#12736);
#3749=VERTEX_POINT('',#12738);
#3750=VERTEX_POINT('',#12742);
#3751=VERTEX_POINT('',#12753);
#3752=VERTEX_POINT('',#12762);
#3753=VERTEX_POINT('',#12764);
#3754=VERTEX_POINT('',#12770);
#3755=VERTEX_POINT('',#12774);
#3756=VERTEX_POINT('',#12776);
#3757=VERTEX_POINT('',#12778);
#3758=VERTEX_POINT('',#12782);
#3759=VERTEX_POINT('',#12784);
#3760=VERTEX_POINT('',#12788);
#3761=VERTEX_POINT('',#12803);
#3762=VERTEX_POINT('',#12808);
#3763=VERTEX_POINT('',#12812);
#3764=VERTEX_POINT('',#12816);
#3765=VERTEX_POINT('',#12820);
#3766=VERTEX_POINT('',#12824);
#3767=VERTEX_POINT('',#12828);
#3768=VERTEX_POINT('',#12835);
#3769=VERTEX_POINT('',#12837);
#3770=VERTEX_POINT('',#12839);
#3771=VERTEX_POINT('',#12841);
#3772=VERTEX_POINT('',#12843);
#3773=VERTEX_POINT('',#12845);
#3774=VERTEX_POINT('',#12847);
#3775=VERTEX_POINT('',#12849);
#3776=VERTEX_POINT('',#12851);
#3777=VERTEX_POINT('',#12853);
#3778=VERTEX_POINT('',#12855);
#3779=VERTEX_POINT('',#12857);
#3780=VERTEX_POINT('',#12859);
#3781=VERTEX_POINT('',#12861);
#3782=VERTEX_POINT('',#12864);
#3783=VERTEX_POINT('',#12865);
#3784=VERTEX_POINT('',#12867);
#3785=VERTEX_POINT('',#12869);
#3786=VERTEX_POINT('',#12871);
#3787=VERTEX_POINT('',#12873);
#3788=VERTEX_POINT('',#12875);
#3789=VERTEX_POINT('',#12877);
#3790=VERTEX_POINT('',#12879);
#3791=VERTEX_POINT('',#12881);
#3792=VERTEX_POINT('',#12884);
#3793=VERTEX_POINT('',#12885);
#3794=VERTEX_POINT('',#12887);
#3795=VERTEX_POINT('',#12889);
#3796=VERTEX_POINT('',#12891);
#3797=VERTEX_POINT('',#12893);
#3798=VERTEX_POINT('',#12895);
#3799=VERTEX_POINT('',#12897);
#3800=VERTEX_POINT('',#12899);
#3801=VERTEX_POINT('',#12901);
#3802=VERTEX_POINT('',#12904);
#3803=VERTEX_POINT('',#12905);
#3804=VERTEX_POINT('',#12909);
#3805=VERTEX_POINT('',#12913);
#3806=VERTEX_POINT('',#12917);
#3807=VERTEX_POINT('',#12921);
#3808=VERTEX_POINT('',#12925);
#3809=VERTEX_POINT('',#12929);
#3810=VERTEX_POINT('',#12933);
#3811=VERTEX_POINT('',#12937);
#3812=VERTEX_POINT('',#12941);
#3813=VERTEX_POINT('',#12948);
#3814=VERTEX_POINT('',#12949);
#3815=VERTEX_POINT('',#12951);
#3816=VERTEX_POINT('',#12953);
#3817=VERTEX_POINT('',#12955);
#3818=VERTEX_POINT('',#12957);
#3819=VERTEX_POINT('',#12959);
#3820=VERTEX_POINT('',#12961);
#3821=VERTEX_POINT('',#12963);
#3822=VERTEX_POINT('',#12965);
#3823=VERTEX_POINT('',#12968);
#3824=VERTEX_POINT('',#12969);
#3825=VERTEX_POINT('',#12973);
#3826=VERTEX_POINT('',#12977);
#3827=VERTEX_POINT('',#12981);
#3828=VERTEX_POINT('',#12985);
#3829=VERTEX_POINT('',#12989);
#3830=VERTEX_POINT('',#12993);
#3831=VERTEX_POINT('',#12997);
#3832=VERTEX_POINT('',#13001);
#3833=VERTEX_POINT('',#13005);
#3834=VERTEX_POINT('',#13012);
#3835=VERTEX_POINT('',#13014);
#3836=VERTEX_POINT('',#13015);
#3837=VERTEX_POINT('',#13019);
#3838=VERTEX_POINT('',#13023);
#3839=VERTEX_POINT('',#13027);
#3840=VERTEX_POINT('',#13031);
#3841=VERTEX_POINT('',#13035);
#3842=VERTEX_POINT('',#13039);
#3843=VERTEX_POINT('',#13043);
#3844=VERTEX_POINT('',#13047);
#3845=VERTEX_POINT('',#13051);
#3846=VERTEX_POINT('',#13058);
#3847=VERTEX_POINT('',#13059);
#3848=VERTEX_POINT('',#13061);
#3849=VERTEX_POINT('',#13063);
#3850=VERTEX_POINT('',#13065);
#3851=VERTEX_POINT('',#13067);
#3852=VERTEX_POINT('',#13069);
#3853=VERTEX_POINT('',#13071);
#3854=VERTEX_POINT('',#13073);
#3855=VERTEX_POINT('',#13075);
#3856=VERTEX_POINT('',#13079);
#3857=VERTEX_POINT('',#13083);
#3858=VERTEX_POINT('',#13085);
#3859=VERTEX_POINT('',#13087);
#3860=VERTEX_POINT('',#13105);
#3861=VERTEX_POINT('',#13110);
#3862=VERTEX_POINT('',#13112);
#3863=VERTEX_POINT('',#13116);
#3864=VERTEX_POINT('',#13120);
#3865=VERTEX_POINT('',#13127);
#3866=VERTEX_POINT('',#13140);
#3867=VERTEX_POINT('',#13144);
#3868=VERTEX_POINT('',#13148);
#3869=VERTEX_POINT('',#13152);
#3870=VERTEX_POINT('',#13156);
#3871=VERTEX_POINT('',#13160);
#3872=VERTEX_POINT('',#13164);
#3873=VERTEX_POINT('',#13172);
#3874=VERTEX_POINT('',#13176);
#3875=VERTEX_POINT('',#13180);
#3876=VERTEX_POINT('',#13184);
#3877=VERTEX_POINT('',#13188);
#3878=VERTEX_POINT('',#13192);
#3879=VERTEX_POINT('',#13199);
#3880=VERTEX_POINT('',#13203);
#3881=VERTEX_POINT('',#13207);
#3882=VERTEX_POINT('',#13211);
#3883=VERTEX_POINT('',#13215);
#3884=VERTEX_POINT('',#13219);
#3885=VERTEX_POINT('',#13275);
#3886=VERTEX_POINT('',#13277);
#3887=VERTEX_POINT('',#13281);
#3888=VERTEX_POINT('',#13285);
#3889=VERTEX_POINT('',#13289);
#3890=VERTEX_POINT('',#13293);
#3891=VERTEX_POINT('',#13297);
#3892=VERTEX_POINT('',#13301);
#3893=VERTEX_POINT('',#13305);
#3894=VERTEX_POINT('',#13309);
#3895=VERTEX_POINT('',#13316);
#3896=VERTEX_POINT('',#13318);
#3897=VERTEX_POINT('',#13322);
#3898=VERTEX_POINT('',#13326);
#3899=VERTEX_POINT('',#13330);
#3900=VERTEX_POINT('',#13334);
#3901=VERTEX_POINT('',#13338);
#3902=VERTEX_POINT('',#13342);
#3903=VERTEX_POINT('',#13346);
#3904=VERTEX_POINT('',#13350);
#3905=VERTEX_POINT('',#13362);
#3906=VERTEX_POINT('',#13364);
#3907=VERTEX_POINT('',#13375);
#3908=VERTEX_POINT('',#13386);
#3909=VERTEX_POINT('',#13397);
#3910=VERTEX_POINT('',#13408);
#3911=VERTEX_POINT('',#13419);
#3912=VERTEX_POINT('',#13430);
#3913=VERTEX_POINT('',#13441);
#3914=VERTEX_POINT('',#13452);
#3915=VERTEX_POINT('',#13463);
#3916=VERTEX_POINT('',#13479);
#3917=VERTEX_POINT('',#13481);
#3918=VERTEX_POINT('',#13485);
#3919=VERTEX_POINT('',#13489);
#3920=VERTEX_POINT('',#13493);
#3921=VERTEX_POINT('',#13497);
#3922=VERTEX_POINT('',#13501);
#3923=VERTEX_POINT('',#13505);
#3924=VERTEX_POINT('',#13509);
#3925=VERTEX_POINT('',#13513);
#3926=VERTEX_POINT('',#13525);
#3927=VERTEX_POINT('',#13527);
#3928=VERTEX_POINT('',#13538);
#3929=VERTEX_POINT('',#13549);
#3930=VERTEX_POINT('',#13560);
#3931=VERTEX_POINT('',#13571);
#3932=VERTEX_POINT('',#13582);
#3933=VERTEX_POINT('',#13593);
#3934=VERTEX_POINT('',#13604);
#3935=VERTEX_POINT('',#13615);
#3936=VERTEX_POINT('',#13626);
#3937=VERTEX_POINT('',#13642);
#3938=VERTEX_POINT('',#13644);
#3939=VERTEX_POINT('',#13648);
#3940=VERTEX_POINT('',#13652);
#3941=VERTEX_POINT('',#13656);
#3942=VERTEX_POINT('',#13660);
#3943=VERTEX_POINT('',#13664);
#3944=VERTEX_POINT('',#13668);
#3945=VERTEX_POINT('',#13672);
#3946=VERTEX_POINT('',#13676);
#3947=VERTEX_POINT('',#13688);
#3948=VERTEX_POINT('',#13690);
#3949=VERTEX_POINT('',#13701);
#3950=VERTEX_POINT('',#13712);
#3951=VERTEX_POINT('',#13723);
#3952=VERTEX_POINT('',#13734);
#3953=VERTEX_POINT('',#13745);
#3954=VERTEX_POINT('',#13756);
#3955=VERTEX_POINT('',#13767);
#3956=VERTEX_POINT('',#13778);
#3957=VERTEX_POINT('',#13789);
#4499=EDGE_CURVE('',#3672,#3673,#1999,.T.);
#4500=EDGE_CURVE('',#3673,#3674,#2000,.T.);
#4501=EDGE_CURVE('',#3674,#3675,#2001,.T.);
#4502=EDGE_CURVE('',#3675,#3672,#2002,.T.);
#4503=EDGE_CURVE('',#3672,#3676,#639,.T.);
#4504=EDGE_CURVE('',#3676,#3677,#2003,.T.);
#4505=EDGE_CURVE('',#3677,#3673,#640,.T.);
#4506=EDGE_CURVE('',#3678,#3679,#2004,.T.);
#4507=EDGE_CURVE('',#3679,#3677,#2005,.T.);
#4508=EDGE_CURVE('',#3676,#3678,#2006,.T.);
#4509=EDGE_CURVE('',#3678,#3680,#641,.T.);
#4510=EDGE_CURVE('',#3680,#3681,#2007,.T.);
#4511=EDGE_CURVE('',#3681,#3679,#642,.T.);
#4512=EDGE_CURVE('',#3682,#3683,#2008,.T.);
#4513=EDGE_CURVE('',#3683,#3681,#2009,.T.);
#4514=EDGE_CURVE('',#3680,#3682,#2010,.T.);
#4515=EDGE_CURVE('',#3682,#3684,#643,.T.);
#4516=EDGE_CURVE('',#3684,#3685,#2011,.T.);
#4517=EDGE_CURVE('',#3685,#3683,#644,.T.);
#4518=EDGE_CURVE('',#3686,#3687,#2012,.T.);
#4519=EDGE_CURVE('',#3687,#3685,#2013,.T.);
#4520=EDGE_CURVE('',#3684,#3686,#2014,.T.);
#4521=EDGE_CURVE('',#3686,#3675,#645,.T.);
#4522=EDGE_CURVE('',#3674,#3687,#646,.T.);
#4523=EDGE_CURVE('',#3678,#3688,#2015,.T.);
#4524=EDGE_CURVE('',#3689,#3688,#647,.T.);
#4525=EDGE_CURVE('',#3689,#3680,#2016,.T.);
#4526=EDGE_CURVE('',#3690,#3676,#2017,.T.);
#4527=EDGE_CURVE('',#3688,#3690,#2018,.T.);
#4528=EDGE_CURVE('',#3672,#3691,#2019,.T.);
#4529=EDGE_CURVE('',#3690,#3691,#648,.T.);
#4530=EDGE_CURVE('',#3692,#3675,#2020,.T.);
#4531=EDGE_CURVE('',#3691,#3692,#2021,.T.);
#4532=EDGE_CURVE('',#3693,#3693,#649,.T.);
#4533=EDGE_CURVE('',#3694,#3694,#650,.T.);
#4534=EDGE_CURVE('',#3695,#3695,#651,.T.);
#4535=EDGE_CURVE('',#3696,#3696,#652,.T.);
#4536=EDGE_CURVE('',#3697,#3697,#653,.T.);
#4537=EDGE_CURVE('',#3689,#3698,#2022,.T.);
#4538=EDGE_CURVE('',#3698,#3699,#2023,.T.);
#4539=EDGE_CURVE('',#3699,#3700,#2024,.T.);
#4540=EDGE_CURVE('',#3700,#3689,#2025,.T.);
#4541=EDGE_CURVE('',#3688,#3701,#2026,.T.);
#4542=EDGE_CURVE('',#3701,#3698,#654,.T.);
#4543=EDGE_CURVE('',#3690,#3702,#2027,.T.);
#4544=EDGE_CURVE('',#3702,#3701,#2028,.T.);
#4545=EDGE_CURVE('',#3691,#3703,#2029,.T.);
#4546=EDGE_CURVE('',#3703,#3702,#655,.T.);
#4547=EDGE_CURVE('',#3692,#3704,#2030,.T.);
#4548=EDGE_CURVE('',#3704,#3703,#2031,.T.);
#4549=EDGE_CURVE('',#3705,#3706,#2032,.T.);
#4550=EDGE_CURVE('',#3706,#3704,#656,.T.);
#4551=EDGE_CURVE('',#3692,#3705,#657,.T.);
#4552=EDGE_CURVE('',#3707,#3708,#188,.T.);
#4553=EDGE_CURVE('',#3708,#3706,#2033,.T.);
#4554=EDGE_CURVE('',#3705,#3709,#2034,.T.);
#4555=EDGE_CURVE('',#3709,#3710,#2035,.T.);
#4556=EDGE_CURVE('',#3710,#3711,#2036,.T.);
#4557=EDGE_CURVE('',#3711,#3712,#189,.T.);
#4558=EDGE_CURVE('',#3712,#3707,#2037,.T.);
#4559=EDGE_CURVE('',#3699,#3710,#658,.T.);
#4560=EDGE_CURVE('',#3709,#3700,#659,.T.);
#4561=EDGE_CURVE('',#3682,#3700,#2038,.T.);
#4562=EDGE_CURVE('',#3713,#3703,#2039,.T.);
#4563=EDGE_CURVE('',#3714,#3713,#660,.T.);
#4564=EDGE_CURVE('',#3714,#3702,#2040,.T.);
#4565=EDGE_CURVE('',#3715,#3704,#2041,.T.);
#4566=EDGE_CURVE('',#3713,#3715,#2042,.T.);
#4567=EDGE_CURVE('',#3716,#3706,#2043,.T.);
#4568=EDGE_CURVE('',#3715,#3716,#661,.T.);
#4569=EDGE_CURVE('',#3717,#3710,#2044,.T.);
#4570=EDGE_CURVE('',#3718,#3717,#2045,.T.);
#4571=EDGE_CURVE('',#3718,#3719,#2046,.T.);
#4572=EDGE_CURVE('',#3719,#3720,#2047,.T.);
#4573=EDGE_CURVE('',#3720,#3721,#2048,.T.);
#4574=EDGE_CURVE('',#3722,#3721,#2049,.T.);
#4575=EDGE_CURVE('',#3722,#3723,#2050,.T.);
#4576=EDGE_CURVE('',#3723,#3724,#2051,.T.);
#4577=EDGE_CURVE('',#3724,#3725,#2052,.T.);
#4578=EDGE_CURVE('',#3725,#3726,#2053,.T.);
#4579=EDGE_CURVE('',#3726,#3727,#190,.T.);
#4580=EDGE_CURVE('',#3711,#3727,#191,.T.);
#4581=EDGE_CURVE('',#3728,#3708,#192,.T.);
#4582=EDGE_CURVE('',#3728,#3729,#193,.T.);
#4583=EDGE_CURVE('',#3716,#3729,#2054,.T.);
#4584=EDGE_CURVE('',#3730,#3707,#194,.F.);
#4585=EDGE_CURVE('',#3730,#3731,#195,.T.);
#4586=EDGE_CURVE('',#3732,#3731,#2055,.T.);
#4587=EDGE_CURVE('',#3733,#3732,#196,.T.);
#4588=EDGE_CURVE('',#3729,#3733,#197,.T.);
#4589=EDGE_CURVE('',#3712,#3734,#198,.F.);
#4590=EDGE_CURVE('',#3734,#3730,#2056,.T.);
#4591=EDGE_CURVE('',#3735,#3735,#662,.T.);
#4592=EDGE_CURVE('',#3735,#3736,#2057,.T.);
#4593=EDGE_CURVE('',#3736,#3737,#663,.T.);
#4594=EDGE_CURVE('',#3737,#3738,#107,.T.);
#4595=EDGE_CURVE('',#3738,#3739,#199,.T.);
#4596=EDGE_CURVE('',#3739,#3740,#108,.T.);
#4597=EDGE_CURVE('',#3740,#3736,#664,.T.);
#4598=EDGE_CURVE('',#3738,#3717,#2058,.T.);
#4599=EDGE_CURVE('',#3717,#3741,#665,.T.);
#4600=EDGE_CURVE('',#3739,#3741,#2059,.T.);
#4601=EDGE_CURVE('',#3737,#3742,#2060,.T.);
#4602=EDGE_CURVE('',#3742,#3743,#2061,.T.);
#4603=EDGE_CURVE('',#3743,#3744,#2062,.T.);
#4604=EDGE_CURVE('',#3744,#3718,#2063,.T.);
#4605=EDGE_CURVE('',#3735,#3745,#2064,.T.);
#4606=EDGE_CURVE('',#3745,#3745,#666,.T.);
#4607=EDGE_CURVE('',#3746,#3746,#667,.T.);
#4608=EDGE_CURVE('',#3746,#3747,#2065,.T.);
#4609=EDGE_CURVE('',#3747,#3748,#668,.T.);
#4610=EDGE_CURVE('',#3748,#3749,#109,.T.);
#4611=EDGE_CURVE('',#3749,#3750,#200,.T.);
#4612=EDGE_CURVE('',#3750,#3751,#110,.T.);
#4613=EDGE_CURVE('',#3751,#3747,#669,.T.);
#4614=EDGE_CURVE('',#3749,#3715,#2066,.T.);
#4615=EDGE_CURVE('',#3750,#3716,#2067,.T.);
#4616=EDGE_CURVE('',#3748,#3752,#2068,.T.);
#4617=EDGE_CURVE('',#3753,#3752,#111,.T.);
#4618=EDGE_CURVE('',#3753,#3713,#2069,.T.);
#4619=EDGE_CURVE('',#3746,#3754,#2070,.T.);
#4620=EDGE_CURVE('',#3754,#3754,#670,.T.);
#4621=EDGE_CURVE('',#3755,#3755,#671,.T.);
#4622=EDGE_CURVE('',#3755,#3756,#2071,.T.);
#4623=EDGE_CURVE('',#3756,#3757,#112,.T.);
#4624=EDGE_CURVE('',#3757,#3758,#672,.T.);
#4625=EDGE_CURVE('',#3758,#3759,#113,.T.);
#4626=EDGE_CURVE('',#3759,#3760,#201,.T.);
#4627=EDGE_CURVE('',#3760,#3756,#114,.T.);
#4628=EDGE_CURVE('',#3741,#3761,#2072,.T.);
#4629=EDGE_CURVE('',#3759,#3761,#2073,.T.);
#4630=EDGE_CURVE('',#3758,#3740,#2074,.T.);
#4631=EDGE_CURVE('',#3762,#3757,#2075,.T.);
#4632=EDGE_CURVE('',#3752,#3762,#673,.T.);
#4633=EDGE_CURVE('',#3733,#3751,#2076,.T.);
#4634=EDGE_CURVE('',#3732,#3763,#202,.T.);
#4635=EDGE_CURVE('',#3763,#3764,#203,.T.);
#4636=EDGE_CURVE('',#3764,#3765,#204,.T.);
#4637=EDGE_CURVE('',#3765,#3766,#205,.T.);
#4638=EDGE_CURVE('',#3766,#3767,#206,.T.);
#4639=EDGE_CURVE('',#3767,#3726,#207,.T.);
#4640=EDGE_CURVE('',#3725,#3768,#2077,.T.);
#4641=EDGE_CURVE('',#3768,#3769,#2078,.T.);
#4642=EDGE_CURVE('',#3769,#3770,#2079,.T.);
#4643=EDGE_CURVE('',#3770,#3771,#2080,.T.);
#4644=EDGE_CURVE('',#3771,#3772,#2081,.T.);
#4645=EDGE_CURVE('',#3772,#3773,#2082,.T.);
#4646=EDGE_CURVE('',#3773,#3774,#2083,.T.);
#4647=EDGE_CURVE('',#3775,#3774,#2084,.T.);
#4648=EDGE_CURVE('',#3775,#3776,#2085,.T.);
#4649=EDGE_CURVE('',#3776,#3777,#2086,.T.);
#4650=EDGE_CURVE('',#3777,#3778,#2087,.T.);
#4651=EDGE_CURVE('',#3778,#3779,#2088,.T.);
#4652=EDGE_CURVE('',#3779,#3780,#2089,.T.);
#4653=EDGE_CURVE('',#3780,#3781,#2090,.T.);
#4654=EDGE_CURVE('',#3781,#3742,#2091,.T.);
#4655=EDGE_CURVE('',#3782,#3783,#2092,.T.);
#4656=EDGE_CURVE('',#3783,#3784,#2093,.T.);
#4657=EDGE_CURVE('',#3784,#3785,#2094,.T.);
#4658=EDGE_CURVE('',#3785,#3786,#2095,.T.);
#4659=EDGE_CURVE('',#3786,#3787,#2096,.T.);
#4660=EDGE_CURVE('',#3787,#3788,#2097,.T.);
#4661=EDGE_CURVE('',#3788,#3789,#2098,.T.);
#4662=EDGE_CURVE('',#3789,#3790,#2099,.T.);
#4663=EDGE_CURVE('',#3790,#3791,#2100,.T.);
#4664=EDGE_CURVE('',#3791,#3782,#2101,.T.);
#4665=EDGE_CURVE('',#3792,#3793,#2102,.T.);
#4666=EDGE_CURVE('',#3793,#3794,#2103,.T.);
#4667=EDGE_CURVE('',#3794,#3795,#2104,.T.);
#4668=EDGE_CURVE('',#3795,#3796,#2105,.T.);
#4669=EDGE_CURVE('',#3796,#3797,#2106,.T.);
#4670=EDGE_CURVE('',#3797,#3798,#2107,.T.);
#4671=EDGE_CURVE('',#3798,#3799,#2108,.T.);
#4672=EDGE_CURVE('',#3799,#3800,#2109,.T.);
#4673=EDGE_CURVE('',#3800,#3801,#2110,.T.);
#4674=EDGE_CURVE('',#3801,#3792,#2111,.T.);
#4675=EDGE_CURVE('',#3802,#3803,#208,.T.);
#4676=EDGE_CURVE('',#3803,#3804,#209,.T.);
#4677=EDGE_CURVE('',#3804,#3805,#210,.T.);
#4678=EDGE_CURVE('',#3805,#3806,#211,.T.);
#4679=EDGE_CURVE('',#3806,#3807,#212,.T.);
#4680=EDGE_CURVE('',#3807,#3808,#213,.T.);
#4681=EDGE_CURVE('',#3808,#3809,#214,.T.);
#4682=EDGE_CURVE('',#3809,#3810,#215,.T.);
#4683=EDGE_CURVE('',#3810,#3811,#216,.T.);
#4684=EDGE_CURVE('',#3811,#3812,#217,.T.);
#4685=EDGE_CURVE('',#3812,#3802,#218,.T.);
#4686=EDGE_CURVE('',#3813,#3814,#2112,.T.);
#4687=EDGE_CURVE('',#3814,#3815,#2113,.T.);
#4688=EDGE_CURVE('',#3815,#3816,#2114,.T.);
#4689=EDGE_CURVE('',#3816,#3817,#2115,.T.);
#4690=EDGE_CURVE('',#3817,#3818,#2116,.T.);
#4691=EDGE_CURVE('',#3818,#3819,#2117,.T.);
#4692=EDGE_CURVE('',#3819,#3820,#2118,.T.);
#4693=EDGE_CURVE('',#3820,#3821,#2119,.T.);
#4694=EDGE_CURVE('',#3821,#3822,#2120,.T.);
#4695=EDGE_CURVE('',#3822,#3813,#2121,.T.);
#4696=EDGE_CURVE('',#3823,#3824,#219,.T.);
#4697=EDGE_CURVE('',#3824,#3825,#220,.T.);
#4698=EDGE_CURVE('',#3825,#3826,#221,.T.);
#4699=EDGE_CURVE('',#3826,#3827,#222,.T.);
#4700=EDGE_CURVE('',#3827,#3828,#223,.T.);
#4701=EDGE_CURVE('',#3828,#3829,#224,.T.);
#4702=EDGE_CURVE('',#3829,#3830,#225,.T.);
#4703=EDGE_CURVE('',#3830,#3831,#226,.T.);
#4704=EDGE_CURVE('',#3831,#3832,#227,.T.);
#4705=EDGE_CURVE('',#3832,#3833,#228,.T.);
#4706=EDGE_CURVE('',#3833,#3823,#229,.T.);
#4707=EDGE_CURVE('',#3834,#3834,#674,.T.);
#4708=EDGE_CURVE('',#3835,#3836,#230,.T.);
#4709=EDGE_CURVE('',#3836,#3837,#231,.T.);
#4710=EDGE_CURVE('',#3837,#3838,#232,.T.);
#4711=EDGE_CURVE('',#3838,#3839,#233,.T.);
#4712=EDGE_CURVE('',#3839,#3840,#234,.T.);
#4713=EDGE_CURVE('',#3840,#3841,#235,.T.);
#4714=EDGE_CURVE('',#3841,#3842,#236,.T.);
#4715=EDGE_CURVE('',#3842,#3843,#237,.T.);
#4716=EDGE_CURVE('',#3843,#3844,#238,.T.);
#4717=EDGE_CURVE('',#3844,#3845,#239,.T.);
#4718=EDGE_CURVE('',#3845,#3835,#240,.T.);
#4719=EDGE_CURVE('',#3846,#3847,#2122,.T.);
#4720=EDGE_CURVE('',#3847,#3848,#2123,.T.);
#4721=EDGE_CURVE('',#3848,#3849,#2124,.T.);
#4722=EDGE_CURVE('',#3849,#3850,#2125,.T.);
#4723=EDGE_CURVE('',#3850,#3851,#2126,.T.);
#4724=EDGE_CURVE('',#3851,#3852,#2127,.T.);
#4725=EDGE_CURVE('',#3852,#3853,#2128,.T.);
#4726=EDGE_CURVE('',#3853,#3854,#2129,.T.);
#4727=EDGE_CURVE('',#3854,#3855,#2130,.T.);
#4728=EDGE_CURVE('',#3855,#3846,#2131,.T.);
#4729=EDGE_CURVE('',#3755,#3856,#2132,.T.);
#4730=EDGE_CURVE('',#3856,#3856,#675,.T.);
#4731=EDGE_CURVE('',#3857,#3857,#676,.T.);
#4732=EDGE_CURVE('',#3857,#3858,#2133,.T.);
#4733=EDGE_CURVE('',#3858,#3859,#115,.T.);
#4734=EDGE_CURVE('',#3859,#3753,#241,.T.);
#4735=EDGE_CURVE('',#3762,#3858,#116,.T.);
#4736=EDGE_CURVE('',#3857,#3860,#2134,.T.);
#4737=EDGE_CURVE('',#3860,#3860,#677,.T.);
#4738=EDGE_CURVE('',#3721,#3775,#2135,.T.);
#4739=EDGE_CURVE('',#3774,#3861,#2136,.T.);
#4740=EDGE_CURVE('',#3861,#3862,#2137,.T.);
#4741=EDGE_CURVE('',#3862,#3722,#2138,.T.);
#4742=EDGE_CURVE('',#3862,#3863,#2139,.T.);
#4743=EDGE_CURVE('',#3863,#3723,#2140,.T.);
#4744=EDGE_CURVE('',#3861,#3864,#2141,.T.);
#4745=EDGE_CURVE('',#3864,#3863,#2142,.T.);
#4746=EDGE_CURVE('',#3859,#3714,#2143,.T.);
#4747=EDGE_CURVE('',#3760,#3865,#2144,.T.);
#4748=EDGE_CURVE('',#3865,#3714,#2145,.T.);
#4749=EDGE_CURVE('',#3761,#3865,#678,.T.);
#4750=EDGE_CURVE('',#3701,#3865,#2146,.T.);
#4751=EDGE_CURVE('',#3761,#3698,#2147,.T.);
#4752=EDGE_CURVE('',#3741,#3699,#2148,.T.);
#4753=EDGE_CURVE('',#3744,#3866,#2149,.T.);
#4754=EDGE_CURVE('',#3866,#3719,#2150,.T.);
#4755=EDGE_CURVE('',#3743,#3867,#2151,.T.);
#4756=EDGE_CURVE('',#3867,#3866,#2152,.T.);
#4757=EDGE_CURVE('',#3868,#3734,#242,.T.);
#4758=EDGE_CURVE('',#3869,#3868,#243,.T.);
#4759=EDGE_CURVE('',#3870,#3869,#244,.T.);
#4760=EDGE_CURVE('',#3871,#3870,#245,.T.);
#4761=EDGE_CURVE('',#3872,#3871,#246,.T.);
#4762=EDGE_CURVE('',#3731,#3872,#247,.T.);
#4763=EDGE_CURVE('',#3781,#3873,#2153,.T.);
#4764=EDGE_CURVE('',#3873,#3867,#2154,.T.);
#4765=EDGE_CURVE('',#3780,#3874,#2155,.T.);
#4766=EDGE_CURVE('',#3874,#3873,#2156,.T.);
#4767=EDGE_CURVE('',#3779,#3875,#2157,.T.);
#4768=EDGE_CURVE('',#3875,#3874,#2158,.T.);
#4769=EDGE_CURVE('',#3778,#3876,#2159,.T.);
#4770=EDGE_CURVE('',#3876,#3875,#2160,.T.);
#4771=EDGE_CURVE('',#3777,#3877,#2161,.T.);
#4772=EDGE_CURVE('',#3877,#3876,#2162,.T.);
#4773=EDGE_CURVE('',#3776,#3878,#2163,.T.);
#4774=EDGE_CURVE('',#3878,#3877,#2164,.T.);
#4775=EDGE_CURVE('',#3720,#3878,#2165,.T.);
#4776=EDGE_CURVE('',#3773,#3879,#2166,.T.);
#4777=EDGE_CURVE('',#3879,#3864,#2167,.T.);
#4778=EDGE_CURVE('',#3772,#3880,#2168,.T.);
#4779=EDGE_CURVE('',#3880,#3879,#2169,.T.);
#4780=EDGE_CURVE('',#3771,#3881,#2170,.T.);
#4781=EDGE_CURVE('',#3881,#3880,#2171,.T.);
#4782=EDGE_CURVE('',#3770,#3882,#2172,.T.);
#4783=EDGE_CURVE('',#3882,#3881,#2173,.T.);
#4784=EDGE_CURVE('',#3769,#3883,#2174,.T.);
#4785=EDGE_CURVE('',#3883,#3882,#2175,.T.);
#4786=EDGE_CURVE('',#3768,#3884,#2176,.T.);
#4787=EDGE_CURVE('',#3884,#3883,#2177,.T.);
#4788=EDGE_CURVE('',#3724,#3884,#2178,.T.);
#4789=EDGE_CURVE('',#3767,#3868,#2179,.T.);
#4790=EDGE_CURVE('',#3766,#3869,#2180,.T.);
#4791=EDGE_CURVE('',#3765,#3870,#2181,.T.);
#4792=EDGE_CURVE('',#3764,#3871,#2182,.T.);
#4793=EDGE_CURVE('',#3763,#3872,#2183,.T.);
#4794=EDGE_CURVE('',#3782,#3885,#2184,.T.);
#4795=EDGE_CURVE('',#3885,#3886,#2185,.T.);
#4796=EDGE_CURVE('',#3783,#3886,#2186,.T.);
#4797=EDGE_CURVE('',#3791,#3887,#2187,.T.);
#4798=EDGE_CURVE('',#3887,#3885,#2188,.T.);
#4799=EDGE_CURVE('',#3790,#3888,#2189,.T.);
#4800=EDGE_CURVE('',#3888,#3887,#2190,.T.);
#4801=EDGE_CURVE('',#3789,#3889,#2191,.T.);
#4802=EDGE_CURVE('',#3889,#3888,#2192,.T.);
#4803=EDGE_CURVE('',#3788,#3890,#2193,.T.);
#4804=EDGE_CURVE('',#3890,#3889,#2194,.T.);
#4805=EDGE_CURVE('',#3787,#3891,#2195,.T.);
#4806=EDGE_CURVE('',#3891,#3890,#2196,.T.);
#4807=EDGE_CURVE('',#3786,#3892,#2197,.T.);
#4808=EDGE_CURVE('',#3892,#3891,#2198,.T.);
#4809=EDGE_CURVE('',#3785,#3893,#2199,.T.);
#4810=EDGE_CURVE('',#3893,#3892,#2200,.T.);
#4811=EDGE_CURVE('',#3784,#3894,#2201,.T.);
#4812=EDGE_CURVE('',#3894,#3893,#2202,.T.);
#4813=EDGE_CURVE('',#3886,#3894,#2203,.T.);
#4814=EDGE_CURVE('',#3792,#3895,#2204,.T.);
#4815=EDGE_CURVE('',#3895,#3896,#2205,.T.);
#4816=EDGE_CURVE('',#3793,#3896,#2206,.T.);
#4817=EDGE_CURVE('',#3801,#3897,#2207,.T.);
#4818=EDGE_CURVE('',#3897,#3895,#2208,.T.);
#4819=EDGE_CURVE('',#3800,#3898,#2209,.T.);
#4820=EDGE_CURVE('',#3898,#3897,#2210,.T.);
#4821=EDGE_CURVE('',#3799,#3899,#2211,.T.);
#4822=EDGE_CURVE('',#3899,#3898,#2212,.T.);
#4823=EDGE_CURVE('',#3798,#3900,#2213,.T.);
#4824=EDGE_CURVE('',#3900,#3899,#2214,.T.);
#4825=EDGE_CURVE('',#3797,#3901,#2215,.T.);
#4826=EDGE_CURVE('',#3901,#3900,#2216,.T.);
#4827=EDGE_CURVE('',#3796,#3902,#2217,.T.);
#4828=EDGE_CURVE('',#3902,#3901,#2218,.T.);
#4829=EDGE_CURVE('',#3795,#3903,#2219,.T.);
#4830=EDGE_CURVE('',#3903,#3902,#2220,.T.);
#4831=EDGE_CURVE('',#3794,#3904,#2221,.T.);
#4832=EDGE_CURVE('',#3904,#3903,#2222,.T.);
#4833=EDGE_CURVE('',#3896,#3904,#2223,.T.);
#4834=EDGE_CURVE('',#3802,#3905,#2224,.T.);
#4835=EDGE_CURVE('',#3905,#3906,#248,.T.);
#4836=EDGE_CURVE('',#3803,#3906,#2225,.T.);
#4837=EDGE_CURVE('',#3812,#3907,#2226,.T.);
#4838=EDGE_CURVE('',#3907,#3905,#249,.T.);
#4839=EDGE_CURVE('',#3811,#3908,#2227,.T.);
#4840=EDGE_CURVE('',#3908,#3907,#250,.T.);
#4841=EDGE_CURVE('',#3810,#3909,#2228,.T.);
#4842=EDGE_CURVE('',#3909,#3908,#251,.T.);
#4843=EDGE_CURVE('',#3809,#3910,#2229,.T.);
#4844=EDGE_CURVE('',#3910,#3909,#252,.T.);
#4845=EDGE_CURVE('',#3808,#3911,#2230,.T.);
#4846=EDGE_CURVE('',#3911,#3910,#253,.T.);
#4847=EDGE_CURVE('',#3807,#3912,#2231,.T.);
#4848=EDGE_CURVE('',#3912,#3911,#254,.T.);
#4849=EDGE_CURVE('',#3806,#3913,#2232,.T.);
#4850=EDGE_CURVE('',#3913,#3912,#255,.T.);
#4851=EDGE_CURVE('',#3805,#3914,#2233,.T.);
#4852=EDGE_CURVE('',#3914,#3913,#256,.T.);
#4853=EDGE_CURVE('',#3804,#3915,#2234,.T.);
#4854=EDGE_CURVE('',#3915,#3914,#257,.T.);
#4855=EDGE_CURVE('',#3906,#3915,#258,.T.);
#4856=EDGE_CURVE('',#3846,#3916,#2235,.T.);
#4857=EDGE_CURVE('',#3916,#3917,#2236,.T.);
#4858=EDGE_CURVE('',#3847,#3917,#2237,.T.);
#4859=EDGE_CURVE('',#3855,#3918,#2238,.T.);
#4860=EDGE_CURVE('',#3918,#3916,#2239,.T.);
#4861=EDGE_CURVE('',#3854,#3919,#2240,.T.);
#4862=EDGE_CURVE('',#3919,#3918,#2241,.T.);
#4863=EDGE_CURVE('',#3853,#3920,#2242,.T.);
#4864=EDGE_CURVE('',#3920,#3919,#2243,.T.);
#4865=EDGE_CURVE('',#3852,#3921,#2244,.T.);
#4866=EDGE_CURVE('',#3921,#3920,#2245,.T.);
#4867=EDGE_CURVE('',#3851,#3922,#2246,.T.);
#4868=EDGE_CURVE('',#3922,#3921,#2247,.T.);
#4869=EDGE_CURVE('',#3850,#3923,#2248,.T.);
#4870=EDGE_CURVE('',#3923,#3922,#2249,.T.);
#4871=EDGE_CURVE('',#3849,#3924,#2250,.T.);
#4872=EDGE_CURVE('',#3924,#3923,#2251,.T.);
#4873=EDGE_CURVE('',#3848,#3925,#2252,.T.);
#4874=EDGE_CURVE('',#3925,#3924,#2253,.T.);
#4875=EDGE_CURVE('',#3917,#3925,#2254,.T.);
#4876=EDGE_CURVE('',#3835,#3926,#2255,.T.);
#4877=EDGE_CURVE('',#3926,#3927,#259,.T.);
#4878=EDGE_CURVE('',#3836,#3927,#2256,.T.);
#4879=EDGE_CURVE('',#3845,#3928,#2257,.T.);
#4880=EDGE_CURVE('',#3928,#3926,#260,.T.);
#4881=EDGE_CURVE('',#3844,#3929,#2258,.T.);
#4882=EDGE_CURVE('',#3929,#3928,#261,.T.);
#4883=EDGE_CURVE('',#3843,#3930,#2259,.T.);
#4884=EDGE_CURVE('',#3930,#3929,#262,.T.);
#4885=EDGE_CURVE('',#3842,#3931,#2260,.T.);
#4886=EDGE_CURVE('',#3931,#3930,#263,.T.);
#4887=EDGE_CURVE('',#3841,#3932,#2261,.T.);
#4888=EDGE_CURVE('',#3932,#3931,#264,.T.);
#4889=EDGE_CURVE('',#3840,#3933,#2262,.T.);
#4890=EDGE_CURVE('',#3933,#3932,#265,.T.);
#4891=EDGE_CURVE('',#3839,#3934,#2263,.T.);
#4892=EDGE_CURVE('',#3934,#3933,#266,.T.);
#4893=EDGE_CURVE('',#3838,#3935,#2264,.T.);
#4894=EDGE_CURVE('',#3935,#3934,#267,.T.);
#4895=EDGE_CURVE('',#3837,#3936,#2265,.T.);
#4896=EDGE_CURVE('',#3936,#3935,#268,.T.);
#4897=EDGE_CURVE('',#3927,#3936,#269,.T.);
#4898=EDGE_CURVE('',#3813,#3937,#2266,.T.);
#4899=EDGE_CURVE('',#3937,#3938,#2267,.T.);
#4900=EDGE_CURVE('',#3814,#3938,#2268,.T.);
#4901=EDGE_CURVE('',#3822,#3939,#2269,.T.);
#4902=EDGE_CURVE('',#3939,#3937,#2270,.T.);
#4903=EDGE_CURVE('',#3821,#3940,#2271,.T.);
#4904=EDGE_CURVE('',#3940,#3939,#2272,.T.);
#4905=EDGE_CURVE('',#3820,#3941,#2273,.T.);
#4906=EDGE_CURVE('',#3941,#3940,#2274,.T.);
#4907=EDGE_CURVE('',#3819,#3942,#2275,.T.);
#4908=EDGE_CURVE('',#3942,#3941,#2276,.T.);
#4909=EDGE_CURVE('',#3818,#3943,#2277,.T.);
#4910=EDGE_CURVE('',#3943,#3942,#2278,.T.);
#4911=EDGE_CURVE('',#3817,#3944,#2279,.T.);
#4912=EDGE_CURVE('',#3944,#3943,#2280,.T.);
#4913=EDGE_CURVE('',#3816,#3945,#2281,.T.);
#4914=EDGE_CURVE('',#3945,#3944,#2282,.T.);
#4915=EDGE_CURVE('',#3815,#3946,#2283,.T.);
#4916=EDGE_CURVE('',#3946,#3945,#2284,.T.);
#4917=EDGE_CURVE('',#3938,#3946,#2285,.T.);
#4918=EDGE_CURVE('',#3823,#3947,#2286,.T.);
#4919=EDGE_CURVE('',#3947,#3948,#270,.T.);
#4920=EDGE_CURVE('',#3824,#3948,#2287,.T.);
#4921=EDGE_CURVE('',#3833,#3949,#2288,.T.);
#4922=EDGE_CURVE('',#3949,#3947,#271,.T.);
#4923=EDGE_CURVE('',#3832,#3950,#2289,.T.);
#4924=EDGE_CURVE('',#3950,#3949,#272,.T.);
#4925=EDGE_CURVE('',#3831,#3951,#2290,.T.);
#4926=EDGE_CURVE('',#3951,#3950,#273,.T.);
#4927=EDGE_CURVE('',#3830,#3952,#2291,.T.);
#4928=EDGE_CURVE('',#3952,#3951,#274,.T.);
#4929=EDGE_CURVE('',#3829,#3953,#2292,.T.);
#4930=EDGE_CURVE('',#3953,#3952,#275,.T.);
#4931=EDGE_CURVE('',#3828,#3954,#2293,.T.);
#4932=EDGE_CURVE('',#3954,#3953,#276,.T.);
#4933=EDGE_CURVE('',#3827,#3955,#2294,.T.);
#4934=EDGE_CURVE('',#3955,#3954,#277,.T.);
#4935=EDGE_CURVE('',#3826,#3956,#2295,.T.);
#4936=EDGE_CURVE('',#3956,#3955,#278,.T.);
#4937=EDGE_CURVE('',#3825,#3957,#2296,.T.);
#4938=EDGE_CURVE('',#3957,#3956,#279,.T.);
#4939=EDGE_CURVE('',#3948,#3957,#280,.T.);
#4940=EDGE_CURVE('',#3860,#3696,#2297,.T.);
#4941=EDGE_CURVE('',#3745,#3695,#2298,.T.);
#4942=EDGE_CURVE('',#3856,#3694,#2299,.T.);
#4943=EDGE_CURVE('',#3754,#3693,#2300,.T.);
#4944=EDGE_CURVE('',#3834,#3697,#2301,.T.);
#4945=EDGE_CURVE('',#3686,#3705,#2302,.T.);
#4946=EDGE_CURVE('',#3709,#3684,#2303,.T.);
#5854=ORIENTED_EDGE('',*,*,#4499,.T.);
#5855=ORIENTED_EDGE('',*,*,#4500,.T.);
#5856=ORIENTED_EDGE('',*,*,#4501,.T.);
#5857=ORIENTED_EDGE('',*,*,#4502,.T.);
#5858=ORIENTED_EDGE('',*,*,#4499,.F.);
#5859=ORIENTED_EDGE('',*,*,#4503,.T.);
#5860=ORIENTED_EDGE('',*,*,#4504,.T.);
#5861=ORIENTED_EDGE('',*,*,#4505,.T.);
#5862=ORIENTED_EDGE('',*,*,#4506,.T.);
#5863=ORIENTED_EDGE('',*,*,#4507,.T.);
#5864=ORIENTED_EDGE('',*,*,#4504,.F.);
#5865=ORIENTED_EDGE('',*,*,#4508,.T.);
#5866=ORIENTED_EDGE('',*,*,#4506,.F.);
#5867=ORIENTED_EDGE('',*,*,#4509,.T.);
#5868=ORIENTED_EDGE('',*,*,#4510,.T.);
#5869=ORIENTED_EDGE('',*,*,#4511,.T.);
#5870=ORIENTED_EDGE('',*,*,#4512,.T.);
#5871=ORIENTED_EDGE('',*,*,#4513,.T.);
#5872=ORIENTED_EDGE('',*,*,#4510,.F.);
#5873=ORIENTED_EDGE('',*,*,#4514,.T.);
#5874=ORIENTED_EDGE('',*,*,#4512,.F.);
#5875=ORIENTED_EDGE('',*,*,#4515,.T.);
#5876=ORIENTED_EDGE('',*,*,#4516,.T.);
#5877=ORIENTED_EDGE('',*,*,#4517,.T.);
#5878=ORIENTED_EDGE('',*,*,#4518,.T.);
#5879=ORIENTED_EDGE('',*,*,#4519,.T.);
#5880=ORIENTED_EDGE('',*,*,#4516,.F.);
#5881=ORIENTED_EDGE('',*,*,#4520,.T.);
#5882=ORIENTED_EDGE('',*,*,#4518,.F.);
#5883=ORIENTED_EDGE('',*,*,#4521,.T.);
#5884=ORIENTED_EDGE('',*,*,#4501,.F.);
#5885=ORIENTED_EDGE('',*,*,#4522,.T.);
#5886=ORIENTED_EDGE('',*,*,#4509,.F.);
#5887=ORIENTED_EDGE('',*,*,#4523,.T.);
#5888=ORIENTED_EDGE('',*,*,#4524,.F.);
#5889=ORIENTED_EDGE('',*,*,#4525,.T.);
#5890=ORIENTED_EDGE('',*,*,#4508,.F.);
#5891=ORIENTED_EDGE('',*,*,#4526,.F.);
#5892=ORIENTED_EDGE('',*,*,#4527,.F.);
#5893=ORIENTED_EDGE('',*,*,#4523,.F.);
#5894=ORIENTED_EDGE('',*,*,#4503,.F.);
#5895=ORIENTED_EDGE('',*,*,#4528,.T.);
#5896=ORIENTED_EDGE('',*,*,#4529,.F.);
#5897=ORIENTED_EDGE('',*,*,#4526,.T.);
#5898=ORIENTED_EDGE('',*,*,#4502,.F.);
#5899=ORIENTED_EDGE('',*,*,#4530,.F.);
#5900=ORIENTED_EDGE('',*,*,#4531,.F.);
#5901=ORIENTED_EDGE('',*,*,#4528,.F.);
#5902=ORIENTED_EDGE('',*,*,#4500,.F.);
#5903=ORIENTED_EDGE('',*,*,#4505,.F.);
#5904=ORIENTED_EDGE('',*,*,#4507,.F.);
#5905=ORIENTED_EDGE('',*,*,#4511,.F.);
#5906=ORIENTED_EDGE('',*,*,#4513,.F.);
#5907=ORIENTED_EDGE('',*,*,#4517,.F.);
#5908=ORIENTED_EDGE('',*,*,#4519,.F.);
#5909=ORIENTED_EDGE('',*,*,#4522,.F.);
#5910=ORIENTED_EDGE('',*,*,#4532,.T.);
#5911=ORIENTED_EDGE('',*,*,#4533,.T.);
#5912=ORIENTED_EDGE('',*,*,#4534,.T.);
#5913=ORIENTED_EDGE('',*,*,#4535,.T.);
#5914=ORIENTED_EDGE('',*,*,#4536,.T.);
#5915=ORIENTED_EDGE('',*,*,#4537,.T.);
#5916=ORIENTED_EDGE('',*,*,#4538,.T.);
#5917=ORIENTED_EDGE('',*,*,#4539,.T.);
#5918=ORIENTED_EDGE('',*,*,#4540,.T.);
#5919=ORIENTED_EDGE('',*,*,#4541,.T.);
#5920=ORIENTED_EDGE('',*,*,#4542,.T.);
#5921=ORIENTED_EDGE('',*,*,#4537,.F.);
#5922=ORIENTED_EDGE('',*,*,#4524,.T.);
#5923=ORIENTED_EDGE('',*,*,#4543,.T.);
#5924=ORIENTED_EDGE('',*,*,#4544,.T.);
#5925=ORIENTED_EDGE('',*,*,#4541,.F.);
#5926=ORIENTED_EDGE('',*,*,#4527,.T.);
#5927=ORIENTED_EDGE('',*,*,#4545,.T.);
#5928=ORIENTED_EDGE('',*,*,#4546,.T.);
#5929=ORIENTED_EDGE('',*,*,#4543,.F.);
#5930=ORIENTED_EDGE('',*,*,#4529,.T.);
#5931=ORIENTED_EDGE('',*,*,#4547,.T.);
#5932=ORIENTED_EDGE('',*,*,#4548,.T.);
#5933=ORIENTED_EDGE('',*,*,#4545,.F.);
#5934=ORIENTED_EDGE('',*,*,#4531,.T.);
#5935=ORIENTED_EDGE('',*,*,#4549,.T.);
#5936=ORIENTED_EDGE('',*,*,#4550,.T.);
#5937=ORIENTED_EDGE('',*,*,#4547,.F.);
#5938=ORIENTED_EDGE('',*,*,#4551,.T.);
#5939=ORIENTED_EDGE('',*,*,#4552,.T.);
#5940=ORIENTED_EDGE('',*,*,#4553,.T.);
#5941=ORIENTED_EDGE('',*,*,#4549,.F.);
#5942=ORIENTED_EDGE('',*,*,#4554,.T.);
#5943=ORIENTED_EDGE('',*,*,#4555,.T.);
#5944=ORIENTED_EDGE('',*,*,#4556,.T.);
#5945=ORIENTED_EDGE('',*,*,#4557,.T.);
#5946=ORIENTED_EDGE('',*,*,#4558,.T.);
#5947=ORIENTED_EDGE('',*,*,#4539,.F.);
#5948=ORIENTED_EDGE('',*,*,#4559,.T.);
#5949=ORIENTED_EDGE('',*,*,#4555,.F.);
#5950=ORIENTED_EDGE('',*,*,#4560,.T.);
#5951=ORIENTED_EDGE('',*,*,#4514,.F.);
#5952=ORIENTED_EDGE('',*,*,#4525,.F.);
#5953=ORIENTED_EDGE('',*,*,#4540,.F.);
#5954=ORIENTED_EDGE('',*,*,#4561,.F.);
#5955=ORIENTED_EDGE('',*,*,#4546,.F.);
#5956=ORIENTED_EDGE('',*,*,#4562,.F.);
#5957=ORIENTED_EDGE('',*,*,#4563,.F.);
#5958=ORIENTED_EDGE('',*,*,#4564,.T.);
#5959=ORIENTED_EDGE('',*,*,#4548,.F.);
#5960=ORIENTED_EDGE('',*,*,#4565,.F.);
#5961=ORIENTED_EDGE('',*,*,#4566,.F.);
#5962=ORIENTED_EDGE('',*,*,#4562,.T.);
#5963=ORIENTED_EDGE('',*,*,#4550,.F.);
#5964=ORIENTED_EDGE('',*,*,#4567,.F.);
#5965=ORIENTED_EDGE('',*,*,#4568,.F.);
#5966=ORIENTED_EDGE('',*,*,#4565,.T.);
#5967=ORIENTED_EDGE('',*,*,#4556,.F.);
#5968=ORIENTED_EDGE('',*,*,#4569,.F.);
#5969=ORIENTED_EDGE('',*,*,#4570,.F.);
#5970=ORIENTED_EDGE('',*,*,#4571,.T.);
#5971=ORIENTED_EDGE('',*,*,#4572,.T.);
#5972=ORIENTED_EDGE('',*,*,#4573,.T.);
#5973=ORIENTED_EDGE('',*,*,#4574,.F.);
#5974=ORIENTED_EDGE('',*,*,#4575,.T.);
#5975=ORIENTED_EDGE('',*,*,#4576,.T.);
#5976=ORIENTED_EDGE('',*,*,#4577,.T.);
#5977=ORIENTED_EDGE('',*,*,#4578,.T.);
#5978=ORIENTED_EDGE('',*,*,#4579,.T.);
#5979=ORIENTED_EDGE('',*,*,#4580,.F.);
#5980=ORIENTED_EDGE('',*,*,#4553,.F.);
#5981=ORIENTED_EDGE('',*,*,#4581,.F.);
#5982=ORIENTED_EDGE('',*,*,#4582,.T.);
#5983=ORIENTED_EDGE('',*,*,#4583,.F.);
#5984=ORIENTED_EDGE('',*,*,#4567,.T.);
#5985=ORIENTED_EDGE('',*,*,#4552,.F.);
#5986=ORIENTED_EDGE('',*,*,#4584,.F.);
#5987=ORIENTED_EDGE('',*,*,#4585,.T.);
#5988=ORIENTED_EDGE('',*,*,#4586,.F.);
#5989=ORIENTED_EDGE('',*,*,#4587,.F.);
#5990=ORIENTED_EDGE('',*,*,#4588,.F.);
#5991=ORIENTED_EDGE('',*,*,#4582,.F.);
#5992=ORIENTED_EDGE('',*,*,#4581,.T.);
#5993=ORIENTED_EDGE('',*,*,#4558,.F.);
#5994=ORIENTED_EDGE('',*,*,#4589,.T.);
#5995=ORIENTED_EDGE('',*,*,#4590,.T.);
#5996=ORIENTED_EDGE('',*,*,#4584,.T.);
#5997=ORIENTED_EDGE('',*,*,#4591,.T.);
#5998=ORIENTED_EDGE('',*,*,#4592,.T.);
#5999=ORIENTED_EDGE('',*,*,#4593,.T.);
#6000=ORIENTED_EDGE('',*,*,#4594,.T.);
#6001=ORIENTED_EDGE('',*,*,#4595,.T.);
#6002=ORIENTED_EDGE('',*,*,#4596,.T.);
#6003=ORIENTED_EDGE('',*,*,#4597,.T.);
#6004=ORIENTED_EDGE('',*,*,#4592,.F.);
#6005=ORIENTED_EDGE('',*,*,#4595,.F.);
#6006=ORIENTED_EDGE('',*,*,#4598,.T.);
#6007=ORIENTED_EDGE('',*,*,#4599,.T.);
#6008=ORIENTED_EDGE('',*,*,#4600,.F.);
#6009=ORIENTED_EDGE('',*,*,#4594,.F.);
#6010=ORIENTED_EDGE('',*,*,#4601,.T.);
#6011=ORIENTED_EDGE('',*,*,#4602,.T.);
#6012=ORIENTED_EDGE('',*,*,#4603,.T.);
#6013=ORIENTED_EDGE('',*,*,#4604,.T.);
#6014=ORIENTED_EDGE('',*,*,#4570,.T.);
#6015=ORIENTED_EDGE('',*,*,#4598,.F.);
#6016=ORIENTED_EDGE('',*,*,#4591,.F.);
#6017=ORIENTED_EDGE('',*,*,#4605,.T.);
#6018=ORIENTED_EDGE('',*,*,#4606,.T.);
#6019=ORIENTED_EDGE('',*,*,#4605,.F.);
#6020=ORIENTED_EDGE('',*,*,#4607,.T.);
#6021=ORIENTED_EDGE('',*,*,#4608,.T.);
#6022=ORIENTED_EDGE('',*,*,#4609,.T.);
#6023=ORIENTED_EDGE('',*,*,#4610,.T.);
#6024=ORIENTED_EDGE('',*,*,#4611,.T.);
#6025=ORIENTED_EDGE('',*,*,#4612,.T.);
#6026=ORIENTED_EDGE('',*,*,#4613,.T.);
#6027=ORIENTED_EDGE('',*,*,#4608,.F.);
#6028=ORIENTED_EDGE('',*,*,#4611,.F.);
#6029=ORIENTED_EDGE('',*,*,#4614,.T.);
#6030=ORIENTED_EDGE('',*,*,#4568,.T.);
#6031=ORIENTED_EDGE('',*,*,#4615,.F.);
#6032=ORIENTED_EDGE('',*,*,#4610,.F.);
#6033=ORIENTED_EDGE('',*,*,#4616,.T.);
#6034=ORIENTED_EDGE('',*,*,#4617,.F.);
#6035=ORIENTED_EDGE('',*,*,#4618,.T.);
#6036=ORIENTED_EDGE('',*,*,#4566,.T.);
#6037=ORIENTED_EDGE('',*,*,#4614,.F.);
#6038=ORIENTED_EDGE('',*,*,#4607,.F.);
#6039=ORIENTED_EDGE('',*,*,#4619,.T.);
#6040=ORIENTED_EDGE('',*,*,#4620,.T.);
#6041=ORIENTED_EDGE('',*,*,#4619,.F.);
#6042=ORIENTED_EDGE('',*,*,#4621,.T.);
#6043=ORIENTED_EDGE('',*,*,#4622,.T.);
#6044=ORIENTED_EDGE('',*,*,#4623,.T.);
#6045=ORIENTED_EDGE('',*,*,#4624,.T.);
#6046=ORIENTED_EDGE('',*,*,#4625,.T.);
#6047=ORIENTED_EDGE('',*,*,#4626,.T.);
#6048=ORIENTED_EDGE('',*,*,#4627,.T.);
#6049=ORIENTED_EDGE('',*,*,#4622,.F.);
#6050=ORIENTED_EDGE('',*,*,#4596,.F.);
#6051=ORIENTED_EDGE('',*,*,#4600,.T.);
#6052=ORIENTED_EDGE('',*,*,#4628,.T.);
#6053=ORIENTED_EDGE('',*,*,#4629,.F.);
#6054=ORIENTED_EDGE('',*,*,#4625,.F.);
#6055=ORIENTED_EDGE('',*,*,#4630,.T.);
#6056=ORIENTED_EDGE('',*,*,#4597,.F.);
#6057=ORIENTED_EDGE('',*,*,#4630,.F.);
#6058=ORIENTED_EDGE('',*,*,#4624,.F.);
#6059=ORIENTED_EDGE('',*,*,#4631,.F.);
#6060=ORIENTED_EDGE('',*,*,#4632,.F.);
#6061=ORIENTED_EDGE('',*,*,#4616,.F.);
#6062=ORIENTED_EDGE('',*,*,#4609,.F.);
#6063=ORIENTED_EDGE('',*,*,#4613,.F.);
#6064=ORIENTED_EDGE('',*,*,#4633,.F.);
#6065=ORIENTED_EDGE('',*,*,#4587,.T.);
#6066=ORIENTED_EDGE('',*,*,#4634,.T.);
#6067=ORIENTED_EDGE('',*,*,#4635,.T.);
#6068=ORIENTED_EDGE('',*,*,#4636,.T.);
#6069=ORIENTED_EDGE('',*,*,#4637,.T.);
#6070=ORIENTED_EDGE('',*,*,#4638,.T.);
#6071=ORIENTED_EDGE('',*,*,#4639,.T.);
#6072=ORIENTED_EDGE('',*,*,#4578,.F.);
#6073=ORIENTED_EDGE('',*,*,#4640,.T.);
#6074=ORIENTED_EDGE('',*,*,#4641,.T.);
#6075=ORIENTED_EDGE('',*,*,#4642,.T.);
#6076=ORIENTED_EDGE('',*,*,#4643,.T.);
#6077=ORIENTED_EDGE('',*,*,#4644,.T.);
#6078=ORIENTED_EDGE('',*,*,#4645,.T.);
#6079=ORIENTED_EDGE('',*,*,#4646,.T.);
#6080=ORIENTED_EDGE('',*,*,#4647,.F.);
#6081=ORIENTED_EDGE('',*,*,#4648,.T.);
#6082=ORIENTED_EDGE('',*,*,#4649,.T.);
#6083=ORIENTED_EDGE('',*,*,#4650,.T.);
#6084=ORIENTED_EDGE('',*,*,#4651,.T.);
#6085=ORIENTED_EDGE('',*,*,#4652,.T.);
#6086=ORIENTED_EDGE('',*,*,#4653,.T.);
#6087=ORIENTED_EDGE('',*,*,#4654,.T.);
#6088=ORIENTED_EDGE('',*,*,#4601,.F.);
#6089=ORIENTED_EDGE('',*,*,#4593,.F.);
#6090=ORIENTED_EDGE('',*,*,#4655,.T.);
#6091=ORIENTED_EDGE('',*,*,#4656,.T.);
#6092=ORIENTED_EDGE('',*,*,#4657,.T.);
#6093=ORIENTED_EDGE('',*,*,#4658,.T.);
#6094=ORIENTED_EDGE('',*,*,#4659,.T.);
#6095=ORIENTED_EDGE('',*,*,#4660,.T.);
#6096=ORIENTED_EDGE('',*,*,#4661,.T.);
#6097=ORIENTED_EDGE('',*,*,#4662,.T.);
#6098=ORIENTED_EDGE('',*,*,#4663,.T.);
#6099=ORIENTED_EDGE('',*,*,#4664,.T.);
#6100=ORIENTED_EDGE('',*,*,#4665,.T.);
#6101=ORIENTED_EDGE('',*,*,#4666,.T.);
#6102=ORIENTED_EDGE('',*,*,#4667,.T.);
#6103=ORIENTED_EDGE('',*,*,#4668,.T.);
#6104=ORIENTED_EDGE('',*,*,#4669,.T.);
#6105=ORIENTED_EDGE('',*,*,#4670,.T.);
#6106=ORIENTED_EDGE('',*,*,#4671,.T.);
#6107=ORIENTED_EDGE('',*,*,#4672,.T.);
#6108=ORIENTED_EDGE('',*,*,#4673,.T.);
#6109=ORIENTED_EDGE('',*,*,#4674,.T.);
#6110=ORIENTED_EDGE('',*,*,#4675,.T.);
#6111=ORIENTED_EDGE('',*,*,#4676,.T.);
#6112=ORIENTED_EDGE('',*,*,#4677,.T.);
#6113=ORIENTED_EDGE('',*,*,#4678,.T.);
#6114=ORIENTED_EDGE('',*,*,#4679,.T.);
#6115=ORIENTED_EDGE('',*,*,#4680,.T.);
#6116=ORIENTED_EDGE('',*,*,#4681,.T.);
#6117=ORIENTED_EDGE('',*,*,#4682,.T.);
#6118=ORIENTED_EDGE('',*,*,#4683,.T.);
#6119=ORIENTED_EDGE('',*,*,#4684,.T.);
#6120=ORIENTED_EDGE('',*,*,#4685,.T.);
#6121=ORIENTED_EDGE('',*,*,#4686,.T.);
#6122=ORIENTED_EDGE('',*,*,#4687,.T.);
#6123=ORIENTED_EDGE('',*,*,#4688,.T.);
#6124=ORIENTED_EDGE('',*,*,#4689,.T.);
#6125=ORIENTED_EDGE('',*,*,#4690,.T.);
#6126=ORIENTED_EDGE('',*,*,#4691,.T.);
#6127=ORIENTED_EDGE('',*,*,#4692,.T.);
#6128=ORIENTED_EDGE('',*,*,#4693,.T.);
#6129=ORIENTED_EDGE('',*,*,#4694,.T.);
#6130=ORIENTED_EDGE('',*,*,#4695,.T.);
#6131=ORIENTED_EDGE('',*,*,#4696,.T.);
#6132=ORIENTED_EDGE('',*,*,#4697,.T.);
#6133=ORIENTED_EDGE('',*,*,#4698,.T.);
#6134=ORIENTED_EDGE('',*,*,#4699,.T.);
#6135=ORIENTED_EDGE('',*,*,#4700,.T.);
#6136=ORIENTED_EDGE('',*,*,#4701,.T.);
#6137=ORIENTED_EDGE('',*,*,#4702,.T.);
#6138=ORIENTED_EDGE('',*,*,#4703,.T.);
#6139=ORIENTED_EDGE('',*,*,#4704,.T.);
#6140=ORIENTED_EDGE('',*,*,#4705,.T.);
#6141=ORIENTED_EDGE('',*,*,#4706,.T.);
#6142=ORIENTED_EDGE('',*,*,#4707,.T.);
#6143=ORIENTED_EDGE('',*,*,#4708,.T.);
#6144=ORIENTED_EDGE('',*,*,#4709,.T.);
#6145=ORIENTED_EDGE('',*,*,#4710,.T.);
#6146=ORIENTED_EDGE('',*,*,#4711,.T.);
#6147=ORIENTED_EDGE('',*,*,#4712,.T.);
#6148=ORIENTED_EDGE('',*,*,#4713,.T.);
#6149=ORIENTED_EDGE('',*,*,#4714,.T.);
#6150=ORIENTED_EDGE('',*,*,#4715,.T.);
#6151=ORIENTED_EDGE('',*,*,#4716,.T.);
#6152=ORIENTED_EDGE('',*,*,#4717,.T.);
#6153=ORIENTED_EDGE('',*,*,#4718,.T.);
#6154=ORIENTED_EDGE('',*,*,#4719,.T.);
#6155=ORIENTED_EDGE('',*,*,#4720,.T.);
#6156=ORIENTED_EDGE('',*,*,#4721,.T.);
#6157=ORIENTED_EDGE('',*,*,#4722,.T.);
#6158=ORIENTED_EDGE('',*,*,#4723,.T.);
#6159=ORIENTED_EDGE('',*,*,#4724,.T.);
#6160=ORIENTED_EDGE('',*,*,#4725,.T.);
#6161=ORIENTED_EDGE('',*,*,#4726,.T.);
#6162=ORIENTED_EDGE('',*,*,#4727,.T.);
#6163=ORIENTED_EDGE('',*,*,#4728,.T.);
#6164=ORIENTED_EDGE('',*,*,#4621,.F.);
#6165=ORIENTED_EDGE('',*,*,#4729,.T.);
#6166=ORIENTED_EDGE('',*,*,#4730,.T.);
#6167=ORIENTED_EDGE('',*,*,#4729,.F.);
#6168=ORIENTED_EDGE('',*,*,#4731,.T.);
#6169=ORIENTED_EDGE('',*,*,#4732,.T.);
#6170=ORIENTED_EDGE('',*,*,#4733,.T.);
#6171=ORIENTED_EDGE('',*,*,#4734,.T.);
#6172=ORIENTED_EDGE('',*,*,#4617,.T.);
#6173=ORIENTED_EDGE('',*,*,#4632,.T.);
#6174=ORIENTED_EDGE('',*,*,#4735,.T.);
#6175=ORIENTED_EDGE('',*,*,#4732,.F.);
#6176=ORIENTED_EDGE('',*,*,#4731,.F.);
#6177=ORIENTED_EDGE('',*,*,#4736,.T.);
#6178=ORIENTED_EDGE('',*,*,#4737,.T.);
#6179=ORIENTED_EDGE('',*,*,#4736,.F.);
#6180=ORIENTED_EDGE('',*,*,#4738,.T.);
#6181=ORIENTED_EDGE('',*,*,#4647,.T.);
#6182=ORIENTED_EDGE('',*,*,#4739,.T.);
#6183=ORIENTED_EDGE('',*,*,#4740,.T.);
#6184=ORIENTED_EDGE('',*,*,#4741,.T.);
#6185=ORIENTED_EDGE('',*,*,#4574,.T.);
#6186=ORIENTED_EDGE('',*,*,#4741,.F.);
#6187=ORIENTED_EDGE('',*,*,#4742,.T.);
#6188=ORIENTED_EDGE('',*,*,#4743,.T.);
#6189=ORIENTED_EDGE('',*,*,#4575,.F.);
#6190=ORIENTED_EDGE('',*,*,#4740,.F.);
#6191=ORIENTED_EDGE('',*,*,#4744,.T.);
#6192=ORIENTED_EDGE('',*,*,#4745,.T.);
#6193=ORIENTED_EDGE('',*,*,#4742,.F.);
#6194=ORIENTED_EDGE('',*,*,#4612,.F.);
#6195=ORIENTED_EDGE('',*,*,#4615,.T.);
#6196=ORIENTED_EDGE('',*,*,#4583,.T.);
#6197=ORIENTED_EDGE('',*,*,#4588,.T.);
#6198=ORIENTED_EDGE('',*,*,#4633,.T.);
#6199=ORIENTED_EDGE('',*,*,#4734,.F.);
#6200=ORIENTED_EDGE('',*,*,#4746,.T.);
#6201=ORIENTED_EDGE('',*,*,#4563,.T.);
#6202=ORIENTED_EDGE('',*,*,#4618,.F.);
#6203=ORIENTED_EDGE('',*,*,#4627,.F.);
#6204=ORIENTED_EDGE('',*,*,#4747,.T.);
#6205=ORIENTED_EDGE('',*,*,#4748,.T.);
#6206=ORIENTED_EDGE('',*,*,#4746,.F.);
#6207=ORIENTED_EDGE('',*,*,#4733,.F.);
#6208=ORIENTED_EDGE('',*,*,#4735,.F.);
#6209=ORIENTED_EDGE('',*,*,#4631,.T.);
#6210=ORIENTED_EDGE('',*,*,#4623,.F.);
#6211=ORIENTED_EDGE('',*,*,#4626,.F.);
#6212=ORIENTED_EDGE('',*,*,#4629,.T.);
#6213=ORIENTED_EDGE('',*,*,#4749,.T.);
#6214=ORIENTED_EDGE('',*,*,#4747,.F.);
#6215=ORIENTED_EDGE('',*,*,#4544,.F.);
#6216=ORIENTED_EDGE('',*,*,#4564,.F.);
#6217=ORIENTED_EDGE('',*,*,#4748,.F.);
#6218=ORIENTED_EDGE('',*,*,#4750,.F.);
#6219=ORIENTED_EDGE('',*,*,#4542,.F.);
#6220=ORIENTED_EDGE('',*,*,#4750,.T.);
#6221=ORIENTED_EDGE('',*,*,#4749,.F.);
#6222=ORIENTED_EDGE('',*,*,#4751,.T.);
#6223=ORIENTED_EDGE('',*,*,#4538,.F.);
#6224=ORIENTED_EDGE('',*,*,#4751,.F.);
#6225=ORIENTED_EDGE('',*,*,#4628,.F.);
#6226=ORIENTED_EDGE('',*,*,#4752,.T.);
#6227=ORIENTED_EDGE('',*,*,#4559,.F.);
#6228=ORIENTED_EDGE('',*,*,#4752,.F.);
#6229=ORIENTED_EDGE('',*,*,#4599,.F.);
#6230=ORIENTED_EDGE('',*,*,#4569,.T.);
#6231=ORIENTED_EDGE('',*,*,#4604,.F.);
#6232=ORIENTED_EDGE('',*,*,#4753,.T.);
#6233=ORIENTED_EDGE('',*,*,#4754,.T.);
#6234=ORIENTED_EDGE('',*,*,#4571,.F.);
#6235=ORIENTED_EDGE('',*,*,#4603,.F.);
#6236=ORIENTED_EDGE('',*,*,#4755,.T.);
#6237=ORIENTED_EDGE('',*,*,#4756,.T.);
#6238=ORIENTED_EDGE('',*,*,#4753,.F.);
#6239=ORIENTED_EDGE('',*,*,#4590,.F.);
#6240=ORIENTED_EDGE('',*,*,#4757,.F.);
#6241=ORIENTED_EDGE('',*,*,#4758,.F.);
#6242=ORIENTED_EDGE('',*,*,#4759,.F.);
#6243=ORIENTED_EDGE('',*,*,#4760,.F.);
#6244=ORIENTED_EDGE('',*,*,#4761,.F.);
#6245=ORIENTED_EDGE('',*,*,#4762,.F.);
#6246=ORIENTED_EDGE('',*,*,#4585,.F.);
#6247=ORIENTED_EDGE('',*,*,#4602,.F.);
#6248=ORIENTED_EDGE('',*,*,#4654,.F.);
#6249=ORIENTED_EDGE('',*,*,#4763,.T.);
#6250=ORIENTED_EDGE('',*,*,#4764,.T.);
#6251=ORIENTED_EDGE('',*,*,#4755,.F.);
#6252=ORIENTED_EDGE('',*,*,#4653,.F.);
#6253=ORIENTED_EDGE('',*,*,#4765,.T.);
#6254=ORIENTED_EDGE('',*,*,#4766,.T.);
#6255=ORIENTED_EDGE('',*,*,#4763,.F.);
#6256=ORIENTED_EDGE('',*,*,#4652,.F.);
#6257=ORIENTED_EDGE('',*,*,#4767,.T.);
#6258=ORIENTED_EDGE('',*,*,#4768,.T.);
#6259=ORIENTED_EDGE('',*,*,#4765,.F.);
#6260=ORIENTED_EDGE('',*,*,#4651,.F.);
#6261=ORIENTED_EDGE('',*,*,#4769,.T.);
#6262=ORIENTED_EDGE('',*,*,#4770,.T.);
#6263=ORIENTED_EDGE('',*,*,#4767,.F.);
#6264=ORIENTED_EDGE('',*,*,#4650,.F.);
#6265=ORIENTED_EDGE('',*,*,#4771,.T.);
#6266=ORIENTED_EDGE('',*,*,#4772,.T.);
#6267=ORIENTED_EDGE('',*,*,#4769,.F.);
#6268=ORIENTED_EDGE('',*,*,#4649,.F.);
#6269=ORIENTED_EDGE('',*,*,#4773,.T.);
#6270=ORIENTED_EDGE('',*,*,#4774,.T.);
#6271=ORIENTED_EDGE('',*,*,#4771,.F.);
#6272=ORIENTED_EDGE('',*,*,#4738,.F.);
#6273=ORIENTED_EDGE('',*,*,#4573,.F.);
#6274=ORIENTED_EDGE('',*,*,#4775,.T.);
#6275=ORIENTED_EDGE('',*,*,#4773,.F.);
#6276=ORIENTED_EDGE('',*,*,#4648,.F.);
#6277=ORIENTED_EDGE('',*,*,#4572,.F.);
#6278=ORIENTED_EDGE('',*,*,#4754,.F.);
#6279=ORIENTED_EDGE('',*,*,#4756,.F.);
#6280=ORIENTED_EDGE('',*,*,#4764,.F.);
#6281=ORIENTED_EDGE('',*,*,#4766,.F.);
#6282=ORIENTED_EDGE('',*,*,#4768,.F.);
#6283=ORIENTED_EDGE('',*,*,#4770,.F.);
#6284=ORIENTED_EDGE('',*,*,#4772,.F.);
#6285=ORIENTED_EDGE('',*,*,#4774,.F.);
#6286=ORIENTED_EDGE('',*,*,#4775,.F.);
#6287=ORIENTED_EDGE('',*,*,#4739,.F.);
#6288=ORIENTED_EDGE('',*,*,#4646,.F.);
#6289=ORIENTED_EDGE('',*,*,#4776,.T.);
#6290=ORIENTED_EDGE('',*,*,#4777,.T.);
#6291=ORIENTED_EDGE('',*,*,#4744,.F.);
#6292=ORIENTED_EDGE('',*,*,#4645,.F.);
#6293=ORIENTED_EDGE('',*,*,#4778,.T.);
#6294=ORIENTED_EDGE('',*,*,#4779,.T.);
#6295=ORIENTED_EDGE('',*,*,#4776,.F.);
#6296=ORIENTED_EDGE('',*,*,#4644,.F.);
#6297=ORIENTED_EDGE('',*,*,#4780,.T.);
#6298=ORIENTED_EDGE('',*,*,#4781,.T.);
#6299=ORIENTED_EDGE('',*,*,#4778,.F.);
#6300=ORIENTED_EDGE('',*,*,#4643,.F.);
#6301=ORIENTED_EDGE('',*,*,#4782,.T.);
#6302=ORIENTED_EDGE('',*,*,#4783,.T.);
#6303=ORIENTED_EDGE('',*,*,#4780,.F.);
#6304=ORIENTED_EDGE('',*,*,#4642,.F.);
#6305=ORIENTED_EDGE('',*,*,#4784,.T.);
#6306=ORIENTED_EDGE('',*,*,#4785,.T.);
#6307=ORIENTED_EDGE('',*,*,#4782,.F.);
#6308=ORIENTED_EDGE('',*,*,#4641,.F.);
#6309=ORIENTED_EDGE('',*,*,#4786,.T.);
#6310=ORIENTED_EDGE('',*,*,#4787,.T.);
#6311=ORIENTED_EDGE('',*,*,#4784,.F.);
#6312=ORIENTED_EDGE('',*,*,#4577,.F.);
#6313=ORIENTED_EDGE('',*,*,#4788,.T.);
#6314=ORIENTED_EDGE('',*,*,#4786,.F.);
#6315=ORIENTED_EDGE('',*,*,#4640,.F.);
#6316=ORIENTED_EDGE('',*,*,#4576,.F.);
#6317=ORIENTED_EDGE('',*,*,#4743,.F.);
#6318=ORIENTED_EDGE('',*,*,#4745,.F.);
#6319=ORIENTED_EDGE('',*,*,#4777,.F.);
#6320=ORIENTED_EDGE('',*,*,#4779,.F.);
#6321=ORIENTED_EDGE('',*,*,#4781,.F.);
#6322=ORIENTED_EDGE('',*,*,#4783,.F.);
#6323=ORIENTED_EDGE('',*,*,#4785,.F.);
#6324=ORIENTED_EDGE('',*,*,#4787,.F.);
#6325=ORIENTED_EDGE('',*,*,#4788,.F.);
#6326=ORIENTED_EDGE('',*,*,#4557,.F.);
#6327=ORIENTED_EDGE('',*,*,#4580,.T.);
#6328=ORIENTED_EDGE('',*,*,#4579,.F.);
#6329=ORIENTED_EDGE('',*,*,#4639,.F.);
#6330=ORIENTED_EDGE('',*,*,#4789,.T.);
#6331=ORIENTED_EDGE('',*,*,#4757,.T.);
#6332=ORIENTED_EDGE('',*,*,#4589,.F.);
#6333=ORIENTED_EDGE('',*,*,#4638,.F.);
#6334=ORIENTED_EDGE('',*,*,#4790,.T.);
#6335=ORIENTED_EDGE('',*,*,#4758,.T.);
#6336=ORIENTED_EDGE('',*,*,#4789,.F.);
#6337=ORIENTED_EDGE('',*,*,#4637,.F.);
#6338=ORIENTED_EDGE('',*,*,#4791,.T.);
#6339=ORIENTED_EDGE('',*,*,#4759,.T.);
#6340=ORIENTED_EDGE('',*,*,#4790,.F.);
#6341=ORIENTED_EDGE('',*,*,#4636,.F.);
#6342=ORIENTED_EDGE('',*,*,#4792,.T.);
#6343=ORIENTED_EDGE('',*,*,#4760,.T.);
#6344=ORIENTED_EDGE('',*,*,#4791,.F.);
#6345=ORIENTED_EDGE('',*,*,#4635,.F.);
#6346=ORIENTED_EDGE('',*,*,#4793,.T.);
#6347=ORIENTED_EDGE('',*,*,#4761,.T.);
#6348=ORIENTED_EDGE('',*,*,#4792,.F.);
#6349=ORIENTED_EDGE('',*,*,#4634,.F.);
#6350=ORIENTED_EDGE('',*,*,#4586,.T.);
#6351=ORIENTED_EDGE('',*,*,#4762,.T.);
#6352=ORIENTED_EDGE('',*,*,#4793,.F.);
#6353=ORIENTED_EDGE('',*,*,#4655,.F.);
#6354=ORIENTED_EDGE('',*,*,#4794,.T.);
#6355=ORIENTED_EDGE('',*,*,#4795,.T.);
#6356=ORIENTED_EDGE('',*,*,#4796,.F.);
#6357=ORIENTED_EDGE('',*,*,#4664,.F.);
#6358=ORIENTED_EDGE('',*,*,#4797,.T.);
#6359=ORIENTED_EDGE('',*,*,#4798,.T.);
#6360=ORIENTED_EDGE('',*,*,#4794,.F.);
#6361=ORIENTED_EDGE('',*,*,#4663,.F.);
#6362=ORIENTED_EDGE('',*,*,#4799,.T.);
#6363=ORIENTED_EDGE('',*,*,#4800,.T.);
#6364=ORIENTED_EDGE('',*,*,#4797,.F.);
#6365=ORIENTED_EDGE('',*,*,#4662,.F.);
#6366=ORIENTED_EDGE('',*,*,#4801,.T.);
#6367=ORIENTED_EDGE('',*,*,#4802,.T.);
#6368=ORIENTED_EDGE('',*,*,#4799,.F.);
#6369=ORIENTED_EDGE('',*,*,#4661,.F.);
#6370=ORIENTED_EDGE('',*,*,#4803,.T.);
#6371=ORIENTED_EDGE('',*,*,#4804,.T.);
#6372=ORIENTED_EDGE('',*,*,#4801,.F.);
#6373=ORIENTED_EDGE('',*,*,#4660,.F.);
#6374=ORIENTED_EDGE('',*,*,#4805,.T.);
#6375=ORIENTED_EDGE('',*,*,#4806,.T.);
#6376=ORIENTED_EDGE('',*,*,#4803,.F.);
#6377=ORIENTED_EDGE('',*,*,#4659,.F.);
#6378=ORIENTED_EDGE('',*,*,#4807,.T.);
#6379=ORIENTED_EDGE('',*,*,#4808,.T.);
#6380=ORIENTED_EDGE('',*,*,#4805,.F.);
#6381=ORIENTED_EDGE('',*,*,#4658,.F.);
#6382=ORIENTED_EDGE('',*,*,#4809,.T.);
#6383=ORIENTED_EDGE('',*,*,#4810,.T.);
#6384=ORIENTED_EDGE('',*,*,#4807,.F.);
#6385=ORIENTED_EDGE('',*,*,#4657,.F.);
#6386=ORIENTED_EDGE('',*,*,#4811,.T.);
#6387=ORIENTED_EDGE('',*,*,#4812,.T.);
#6388=ORIENTED_EDGE('',*,*,#4809,.F.);
#6389=ORIENTED_EDGE('',*,*,#4656,.F.);
#6390=ORIENTED_EDGE('',*,*,#4796,.T.);
#6391=ORIENTED_EDGE('',*,*,#4813,.T.);
#6392=ORIENTED_EDGE('',*,*,#4811,.F.);
#6393=ORIENTED_EDGE('',*,*,#4813,.F.);
#6394=ORIENTED_EDGE('',*,*,#4795,.F.);
#6395=ORIENTED_EDGE('',*,*,#4798,.F.);
#6396=ORIENTED_EDGE('',*,*,#4800,.F.);
#6397=ORIENTED_EDGE('',*,*,#4802,.F.);
#6398=ORIENTED_EDGE('',*,*,#4804,.F.);
#6399=ORIENTED_EDGE('',*,*,#4806,.F.);
#6400=ORIENTED_EDGE('',*,*,#4808,.F.);
#6401=ORIENTED_EDGE('',*,*,#4810,.F.);
#6402=ORIENTED_EDGE('',*,*,#4812,.F.);
#6403=ORIENTED_EDGE('',*,*,#4665,.F.);
#6404=ORIENTED_EDGE('',*,*,#4814,.T.);
#6405=ORIENTED_EDGE('',*,*,#4815,.T.);
#6406=ORIENTED_EDGE('',*,*,#4816,.F.);
#6407=ORIENTED_EDGE('',*,*,#4674,.F.);
#6408=ORIENTED_EDGE('',*,*,#4817,.T.);
#6409=ORIENTED_EDGE('',*,*,#4818,.T.);
#6410=ORIENTED_EDGE('',*,*,#4814,.F.);
#6411=ORIENTED_EDGE('',*,*,#4673,.F.);
#6412=ORIENTED_EDGE('',*,*,#4819,.T.);
#6413=ORIENTED_EDGE('',*,*,#4820,.T.);
#6414=ORIENTED_EDGE('',*,*,#4817,.F.);
#6415=ORIENTED_EDGE('',*,*,#4672,.F.);
#6416=ORIENTED_EDGE('',*,*,#4821,.T.);
#6417=ORIENTED_EDGE('',*,*,#4822,.T.);
#6418=ORIENTED_EDGE('',*,*,#4819,.F.);
#6419=ORIENTED_EDGE('',*,*,#4671,.F.);
#6420=ORIENTED_EDGE('',*,*,#4823,.T.);
#6421=ORIENTED_EDGE('',*,*,#4824,.T.);
#6422=ORIENTED_EDGE('',*,*,#4821,.F.);
#6423=ORIENTED_EDGE('',*,*,#4670,.F.);
#6424=ORIENTED_EDGE('',*,*,#4825,.T.);
#6425=ORIENTED_EDGE('',*,*,#4826,.T.);
#6426=ORIENTED_EDGE('',*,*,#4823,.F.);
#6427=ORIENTED_EDGE('',*,*,#4669,.F.);
#6428=ORIENTED_EDGE('',*,*,#4827,.T.);
#6429=ORIENTED_EDGE('',*,*,#4828,.T.);
#6430=ORIENTED_EDGE('',*,*,#4825,.F.);
#6431=ORIENTED_EDGE('',*,*,#4668,.F.);
#6432=ORIENTED_EDGE('',*,*,#4829,.T.);
#6433=ORIENTED_EDGE('',*,*,#4830,.T.);
#6434=ORIENTED_EDGE('',*,*,#4827,.F.);
#6435=ORIENTED_EDGE('',*,*,#4667,.F.);
#6436=ORIENTED_EDGE('',*,*,#4831,.T.);
#6437=ORIENTED_EDGE('',*,*,#4832,.T.);
#6438=ORIENTED_EDGE('',*,*,#4829,.F.);
#6439=ORIENTED_EDGE('',*,*,#4666,.F.);
#6440=ORIENTED_EDGE('',*,*,#4816,.T.);
#6441=ORIENTED_EDGE('',*,*,#4833,.T.);
#6442=ORIENTED_EDGE('',*,*,#4831,.F.);
#6443=ORIENTED_EDGE('',*,*,#4833,.F.);
#6444=ORIENTED_EDGE('',*,*,#4815,.F.);
#6445=ORIENTED_EDGE('',*,*,#4818,.F.);
#6446=ORIENTED_EDGE('',*,*,#4820,.F.);
#6447=ORIENTED_EDGE('',*,*,#4822,.F.);
#6448=ORIENTED_EDGE('',*,*,#4824,.F.);
#6449=ORIENTED_EDGE('',*,*,#4826,.F.);
#6450=ORIENTED_EDGE('',*,*,#4828,.F.);
#6451=ORIENTED_EDGE('',*,*,#4830,.F.);
#6452=ORIENTED_EDGE('',*,*,#4832,.F.);
#6453=ORIENTED_EDGE('',*,*,#4675,.F.);
#6454=ORIENTED_EDGE('',*,*,#4834,.T.);
#6455=ORIENTED_EDGE('',*,*,#4835,.T.);
#6456=ORIENTED_EDGE('',*,*,#4836,.F.);
#6457=ORIENTED_EDGE('',*,*,#4685,.F.);
#6458=ORIENTED_EDGE('',*,*,#4837,.T.);
#6459=ORIENTED_EDGE('',*,*,#4838,.T.);
#6460=ORIENTED_EDGE('',*,*,#4834,.F.);
#6461=ORIENTED_EDGE('',*,*,#4684,.F.);
#6462=ORIENTED_EDGE('',*,*,#4839,.T.);
#6463=ORIENTED_EDGE('',*,*,#4840,.T.);
#6464=ORIENTED_EDGE('',*,*,#4837,.F.);
#6465=ORIENTED_EDGE('',*,*,#4683,.F.);
#6466=ORIENTED_EDGE('',*,*,#4841,.T.);
#6467=ORIENTED_EDGE('',*,*,#4842,.T.);
#6468=ORIENTED_EDGE('',*,*,#4839,.F.);
#6469=ORIENTED_EDGE('',*,*,#4682,.F.);
#6470=ORIENTED_EDGE('',*,*,#4843,.T.);
#6471=ORIENTED_EDGE('',*,*,#4844,.T.);
#6472=ORIENTED_EDGE('',*,*,#4841,.F.);
#6473=ORIENTED_EDGE('',*,*,#4681,.F.);
#6474=ORIENTED_EDGE('',*,*,#4845,.T.);
#6475=ORIENTED_EDGE('',*,*,#4846,.T.);
#6476=ORIENTED_EDGE('',*,*,#4843,.F.);
#6477=ORIENTED_EDGE('',*,*,#4680,.F.);
#6478=ORIENTED_EDGE('',*,*,#4847,.T.);
#6479=ORIENTED_EDGE('',*,*,#4848,.T.);
#6480=ORIENTED_EDGE('',*,*,#4845,.F.);
#6481=ORIENTED_EDGE('',*,*,#4679,.F.);
#6482=ORIENTED_EDGE('',*,*,#4849,.T.);
#6483=ORIENTED_EDGE('',*,*,#4850,.T.);
#6484=ORIENTED_EDGE('',*,*,#4847,.F.);
#6485=ORIENTED_EDGE('',*,*,#4678,.F.);
#6486=ORIENTED_EDGE('',*,*,#4851,.T.);
#6487=ORIENTED_EDGE('',*,*,#4852,.T.);
#6488=ORIENTED_EDGE('',*,*,#4849,.F.);
#6489=ORIENTED_EDGE('',*,*,#4677,.F.);
#6490=ORIENTED_EDGE('',*,*,#4853,.T.);
#6491=ORIENTED_EDGE('',*,*,#4854,.T.);
#6492=ORIENTED_EDGE('',*,*,#4851,.F.);
#6493=ORIENTED_EDGE('',*,*,#4676,.F.);
#6494=ORIENTED_EDGE('',*,*,#4836,.T.);
#6495=ORIENTED_EDGE('',*,*,#4855,.T.);
#6496=ORIENTED_EDGE('',*,*,#4853,.F.);
#6497=ORIENTED_EDGE('',*,*,#4855,.F.);
#6498=ORIENTED_EDGE('',*,*,#4835,.F.);
#6499=ORIENTED_EDGE('',*,*,#4838,.F.);
#6500=ORIENTED_EDGE('',*,*,#4840,.F.);
#6501=ORIENTED_EDGE('',*,*,#4842,.F.);
#6502=ORIENTED_EDGE('',*,*,#4844,.F.);
#6503=ORIENTED_EDGE('',*,*,#4846,.F.);
#6504=ORIENTED_EDGE('',*,*,#4848,.F.);
#6505=ORIENTED_EDGE('',*,*,#4850,.F.);
#6506=ORIENTED_EDGE('',*,*,#4852,.F.);
#6507=ORIENTED_EDGE('',*,*,#4854,.F.);
#6508=ORIENTED_EDGE('',*,*,#4719,.F.);
#6509=ORIENTED_EDGE('',*,*,#4856,.T.);
#6510=ORIENTED_EDGE('',*,*,#4857,.T.);
#6511=ORIENTED_EDGE('',*,*,#4858,.F.);
#6512=ORIENTED_EDGE('',*,*,#4728,.F.);
#6513=ORIENTED_EDGE('',*,*,#4859,.T.);
#6514=ORIENTED_EDGE('',*,*,#4860,.T.);
#6515=ORIENTED_EDGE('',*,*,#4856,.F.);
#6516=ORIENTED_EDGE('',*,*,#4727,.F.);
#6517=ORIENTED_EDGE('',*,*,#4861,.T.);
#6518=ORIENTED_EDGE('',*,*,#4862,.T.);
#6519=ORIENTED_EDGE('',*,*,#4859,.F.);
#6520=ORIENTED_EDGE('',*,*,#4726,.F.);
#6521=ORIENTED_EDGE('',*,*,#4863,.T.);
#6522=ORIENTED_EDGE('',*,*,#4864,.T.);
#6523=ORIENTED_EDGE('',*,*,#4861,.F.);
#6524=ORIENTED_EDGE('',*,*,#4725,.F.);
#6525=ORIENTED_EDGE('',*,*,#4865,.T.);
#6526=ORIENTED_EDGE('',*,*,#4866,.T.);
#6527=ORIENTED_EDGE('',*,*,#4863,.F.);
#6528=ORIENTED_EDGE('',*,*,#4724,.F.);
#6529=ORIENTED_EDGE('',*,*,#4867,.T.);
#6530=ORIENTED_EDGE('',*,*,#4868,.T.);
#6531=ORIENTED_EDGE('',*,*,#4865,.F.);
#6532=ORIENTED_EDGE('',*,*,#4723,.F.);
#6533=ORIENTED_EDGE('',*,*,#4869,.T.);
#6534=ORIENTED_EDGE('',*,*,#4870,.T.);
#6535=ORIENTED_EDGE('',*,*,#4867,.F.);
#6536=ORIENTED_EDGE('',*,*,#4722,.F.);
#6537=ORIENTED_EDGE('',*,*,#4871,.T.);
#6538=ORIENTED_EDGE('',*,*,#4872,.T.);
#6539=ORIENTED_EDGE('',*,*,#4869,.F.);
#6540=ORIENTED_EDGE('',*,*,#4721,.F.);
#6541=ORIENTED_EDGE('',*,*,#4873,.T.);
#6542=ORIENTED_EDGE('',*,*,#4874,.T.);
#6543=ORIENTED_EDGE('',*,*,#4871,.F.);
#6544=ORIENTED_EDGE('',*,*,#4720,.F.);
#6545=ORIENTED_EDGE('',*,*,#4858,.T.);
#6546=ORIENTED_EDGE('',*,*,#4875,.T.);
#6547=ORIENTED_EDGE('',*,*,#4873,.F.);
#6548=ORIENTED_EDGE('',*,*,#4875,.F.);
#6549=ORIENTED_EDGE('',*,*,#4857,.F.);
#6550=ORIENTED_EDGE('',*,*,#4860,.F.);
#6551=ORIENTED_EDGE('',*,*,#4862,.F.);
#6552=ORIENTED_EDGE('',*,*,#4864,.F.);
#6553=ORIENTED_EDGE('',*,*,#4866,.F.);
#6554=ORIENTED_EDGE('',*,*,#4868,.F.);
#6555=ORIENTED_EDGE('',*,*,#4870,.F.);
#6556=ORIENTED_EDGE('',*,*,#4872,.F.);
#6557=ORIENTED_EDGE('',*,*,#4874,.F.);
#6558=ORIENTED_EDGE('',*,*,#4708,.F.);
#6559=ORIENTED_EDGE('',*,*,#4876,.T.);
#6560=ORIENTED_EDGE('',*,*,#4877,.T.);
#6561=ORIENTED_EDGE('',*,*,#4878,.F.);
#6562=ORIENTED_EDGE('',*,*,#4718,.F.);
#6563=ORIENTED_EDGE('',*,*,#4879,.T.);
#6564=ORIENTED_EDGE('',*,*,#4880,.T.);
#6565=ORIENTED_EDGE('',*,*,#4876,.F.);
#6566=ORIENTED_EDGE('',*,*,#4717,.F.);
#6567=ORIENTED_EDGE('',*,*,#4881,.T.);
#6568=ORIENTED_EDGE('',*,*,#4882,.T.);
#6569=ORIENTED_EDGE('',*,*,#4879,.F.);
#6570=ORIENTED_EDGE('',*,*,#4716,.F.);
#6571=ORIENTED_EDGE('',*,*,#4883,.T.);
#6572=ORIENTED_EDGE('',*,*,#4884,.T.);
#6573=ORIENTED_EDGE('',*,*,#4881,.F.);
#6574=ORIENTED_EDGE('',*,*,#4715,.F.);
#6575=ORIENTED_EDGE('',*,*,#4885,.T.);
#6576=ORIENTED_EDGE('',*,*,#4886,.T.);
#6577=ORIENTED_EDGE('',*,*,#4883,.F.);
#6578=ORIENTED_EDGE('',*,*,#4714,.F.);
#6579=ORIENTED_EDGE('',*,*,#4887,.T.);
#6580=ORIENTED_EDGE('',*,*,#4888,.T.);
#6581=ORIENTED_EDGE('',*,*,#4885,.F.);
#6582=ORIENTED_EDGE('',*,*,#4713,.F.);
#6583=ORIENTED_EDGE('',*,*,#4889,.T.);
#6584=ORIENTED_EDGE('',*,*,#4890,.T.);
#6585=ORIENTED_EDGE('',*,*,#4887,.F.);
#6586=ORIENTED_EDGE('',*,*,#4712,.F.);
#6587=ORIENTED_EDGE('',*,*,#4891,.T.);
#6588=ORIENTED_EDGE('',*,*,#4892,.T.);
#6589=ORIENTED_EDGE('',*,*,#4889,.F.);
#6590=ORIENTED_EDGE('',*,*,#4711,.F.);
#6591=ORIENTED_EDGE('',*,*,#4893,.T.);
#6592=ORIENTED_EDGE('',*,*,#4894,.T.);
#6593=ORIENTED_EDGE('',*,*,#4891,.F.);
#6594=ORIENTED_EDGE('',*,*,#4710,.F.);
#6595=ORIENTED_EDGE('',*,*,#4895,.T.);
#6596=ORIENTED_EDGE('',*,*,#4896,.T.);
#6597=ORIENTED_EDGE('',*,*,#4893,.F.);
#6598=ORIENTED_EDGE('',*,*,#4709,.F.);
#6599=ORIENTED_EDGE('',*,*,#4878,.T.);
#6600=ORIENTED_EDGE('',*,*,#4897,.T.);
#6601=ORIENTED_EDGE('',*,*,#4895,.F.);
#6602=ORIENTED_EDGE('',*,*,#4897,.F.);
#6603=ORIENTED_EDGE('',*,*,#4877,.F.);
#6604=ORIENTED_EDGE('',*,*,#4880,.F.);
#6605=ORIENTED_EDGE('',*,*,#4882,.F.);
#6606=ORIENTED_EDGE('',*,*,#4884,.F.);
#6607=ORIENTED_EDGE('',*,*,#4886,.F.);
#6608=ORIENTED_EDGE('',*,*,#4888,.F.);
#6609=ORIENTED_EDGE('',*,*,#4890,.F.);
#6610=ORIENTED_EDGE('',*,*,#4892,.F.);
#6611=ORIENTED_EDGE('',*,*,#4894,.F.);
#6612=ORIENTED_EDGE('',*,*,#4896,.F.);
#6613=ORIENTED_EDGE('',*,*,#4686,.F.);
#6614=ORIENTED_EDGE('',*,*,#4898,.T.);
#6615=ORIENTED_EDGE('',*,*,#4899,.T.);
#6616=ORIENTED_EDGE('',*,*,#4900,.F.);
#6617=ORIENTED_EDGE('',*,*,#4695,.F.);
#6618=ORIENTED_EDGE('',*,*,#4901,.T.);
#6619=ORIENTED_EDGE('',*,*,#4902,.T.);
#6620=ORIENTED_EDGE('',*,*,#4898,.F.);
#6621=ORIENTED_EDGE('',*,*,#4694,.F.);
#6622=ORIENTED_EDGE('',*,*,#4903,.T.);
#6623=ORIENTED_EDGE('',*,*,#4904,.T.);
#6624=ORIENTED_EDGE('',*,*,#4901,.F.);
#6625=ORIENTED_EDGE('',*,*,#4693,.F.);
#6626=ORIENTED_EDGE('',*,*,#4905,.T.);
#6627=ORIENTED_EDGE('',*,*,#4906,.T.);
#6628=ORIENTED_EDGE('',*,*,#4903,.F.);
#6629=ORIENTED_EDGE('',*,*,#4692,.F.);
#6630=ORIENTED_EDGE('',*,*,#4907,.T.);
#6631=ORIENTED_EDGE('',*,*,#4908,.T.);
#6632=ORIENTED_EDGE('',*,*,#4905,.F.);
#6633=ORIENTED_EDGE('',*,*,#4691,.F.);
#6634=ORIENTED_EDGE('',*,*,#4909,.T.);
#6635=ORIENTED_EDGE('',*,*,#4910,.T.);
#6636=ORIENTED_EDGE('',*,*,#4907,.F.);
#6637=ORIENTED_EDGE('',*,*,#4690,.F.);
#6638=ORIENTED_EDGE('',*,*,#4911,.T.);
#6639=ORIENTED_EDGE('',*,*,#4912,.T.);
#6640=ORIENTED_EDGE('',*,*,#4909,.F.);
#6641=ORIENTED_EDGE('',*,*,#4689,.F.);
#6642=ORIENTED_EDGE('',*,*,#4913,.T.);
#6643=ORIENTED_EDGE('',*,*,#4914,.T.);
#6644=ORIENTED_EDGE('',*,*,#4911,.F.);
#6645=ORIENTED_EDGE('',*,*,#4688,.F.);
#6646=ORIENTED_EDGE('',*,*,#4915,.T.);
#6647=ORIENTED_EDGE('',*,*,#4916,.T.);
#6648=ORIENTED_EDGE('',*,*,#4913,.F.);
#6649=ORIENTED_EDGE('',*,*,#4687,.F.);
#6650=ORIENTED_EDGE('',*,*,#4900,.T.);
#6651=ORIENTED_EDGE('',*,*,#4917,.T.);
#6652=ORIENTED_EDGE('',*,*,#4915,.F.);
#6653=ORIENTED_EDGE('',*,*,#4917,.F.);
#6654=ORIENTED_EDGE('',*,*,#4899,.F.);
#6655=ORIENTED_EDGE('',*,*,#4902,.F.);
#6656=ORIENTED_EDGE('',*,*,#4904,.F.);
#6657=ORIENTED_EDGE('',*,*,#4906,.F.);
#6658=ORIENTED_EDGE('',*,*,#4908,.F.);
#6659=ORIENTED_EDGE('',*,*,#4910,.F.);
#6660=ORIENTED_EDGE('',*,*,#4912,.F.);
#6661=ORIENTED_EDGE('',*,*,#4914,.F.);
#6662=ORIENTED_EDGE('',*,*,#4916,.F.);
#6663=ORIENTED_EDGE('',*,*,#4696,.F.);
#6664=ORIENTED_EDGE('',*,*,#4918,.T.);
#6665=ORIENTED_EDGE('',*,*,#4919,.T.);
#6666=ORIENTED_EDGE('',*,*,#4920,.F.);
#6667=ORIENTED_EDGE('',*,*,#4706,.F.);
#6668=ORIENTED_EDGE('',*,*,#4921,.T.);
#6669=ORIENTED_EDGE('',*,*,#4922,.T.);
#6670=ORIENTED_EDGE('',*,*,#4918,.F.);
#6671=ORIENTED_EDGE('',*,*,#4705,.F.);
#6672=ORIENTED_EDGE('',*,*,#4923,.T.);
#6673=ORIENTED_EDGE('',*,*,#4924,.T.);
#6674=ORIENTED_EDGE('',*,*,#4921,.F.);
#6675=ORIENTED_EDGE('',*,*,#4704,.F.);
#6676=ORIENTED_EDGE('',*,*,#4925,.T.);
#6677=ORIENTED_EDGE('',*,*,#4926,.T.);
#6678=ORIENTED_EDGE('',*,*,#4923,.F.);
#6679=ORIENTED_EDGE('',*,*,#4703,.F.);
#6680=ORIENTED_EDGE('',*,*,#4927,.T.);
#6681=ORIENTED_EDGE('',*,*,#4928,.T.);
#6682=ORIENTED_EDGE('',*,*,#4925,.F.);
#6683=ORIENTED_EDGE('',*,*,#4702,.F.);
#6684=ORIENTED_EDGE('',*,*,#4929,.T.);
#6685=ORIENTED_EDGE('',*,*,#4930,.T.);
#6686=ORIENTED_EDGE('',*,*,#4927,.F.);
#6687=ORIENTED_EDGE('',*,*,#4701,.F.);
#6688=ORIENTED_EDGE('',*,*,#4931,.T.);
#6689=ORIENTED_EDGE('',*,*,#4932,.T.);
#6690=ORIENTED_EDGE('',*,*,#4929,.F.);
#6691=ORIENTED_EDGE('',*,*,#4700,.F.);
#6692=ORIENTED_EDGE('',*,*,#4933,.T.);
#6693=ORIENTED_EDGE('',*,*,#4934,.T.);
#6694=ORIENTED_EDGE('',*,*,#4931,.F.);
#6695=ORIENTED_EDGE('',*,*,#4699,.F.);
#6696=ORIENTED_EDGE('',*,*,#4935,.T.);
#6697=ORIENTED_EDGE('',*,*,#4936,.T.);
#6698=ORIENTED_EDGE('',*,*,#4933,.F.);
#6699=ORIENTED_EDGE('',*,*,#4698,.F.);
#6700=ORIENTED_EDGE('',*,*,#4937,.T.);
#6701=ORIENTED_EDGE('',*,*,#4938,.T.);
#6702=ORIENTED_EDGE('',*,*,#4935,.F.);
#6703=ORIENTED_EDGE('',*,*,#4697,.F.);
#6704=ORIENTED_EDGE('',*,*,#4920,.T.);
#6705=ORIENTED_EDGE('',*,*,#4939,.T.);
#6706=ORIENTED_EDGE('',*,*,#4937,.F.);
#6707=ORIENTED_EDGE('',*,*,#4939,.F.);
#6708=ORIENTED_EDGE('',*,*,#4919,.F.);
#6709=ORIENTED_EDGE('',*,*,#4922,.F.);
#6710=ORIENTED_EDGE('',*,*,#4924,.F.);
#6711=ORIENTED_EDGE('',*,*,#4926,.F.);
#6712=ORIENTED_EDGE('',*,*,#4928,.F.);
#6713=ORIENTED_EDGE('',*,*,#4930,.F.);
#6714=ORIENTED_EDGE('',*,*,#4932,.F.);
#6715=ORIENTED_EDGE('',*,*,#4934,.F.);
#6716=ORIENTED_EDGE('',*,*,#4936,.F.);
#6717=ORIENTED_EDGE('',*,*,#4938,.F.);
#6718=ORIENTED_EDGE('',*,*,#4737,.F.);
#6719=ORIENTED_EDGE('',*,*,#4940,.T.);
#6720=ORIENTED_EDGE('',*,*,#4535,.F.);
#6721=ORIENTED_EDGE('',*,*,#4940,.F.);
#6722=ORIENTED_EDGE('',*,*,#4606,.F.);
#6723=ORIENTED_EDGE('',*,*,#4941,.T.);
#6724=ORIENTED_EDGE('',*,*,#4534,.F.);
#6725=ORIENTED_EDGE('',*,*,#4941,.F.);
#6726=ORIENTED_EDGE('',*,*,#4730,.F.);
#6727=ORIENTED_EDGE('',*,*,#4942,.T.);
#6728=ORIENTED_EDGE('',*,*,#4533,.F.);
#6729=ORIENTED_EDGE('',*,*,#4942,.F.);
#6730=ORIENTED_EDGE('',*,*,#4620,.F.);
#6731=ORIENTED_EDGE('',*,*,#4943,.T.);
#6732=ORIENTED_EDGE('',*,*,#4532,.F.);
#6733=ORIENTED_EDGE('',*,*,#4943,.F.);
#6734=ORIENTED_EDGE('',*,*,#4707,.F.);
#6735=ORIENTED_EDGE('',*,*,#4944,.T.);
#6736=ORIENTED_EDGE('',*,*,#4536,.F.);
#6737=ORIENTED_EDGE('',*,*,#4944,.F.);
#6738=ORIENTED_EDGE('',*,*,#4521,.F.);
#6739=ORIENTED_EDGE('',*,*,#4945,.T.);
#6740=ORIENTED_EDGE('',*,*,#4551,.F.);
#6741=ORIENTED_EDGE('',*,*,#4530,.T.);
#6742=ORIENTED_EDGE('',*,*,#4515,.F.);
#6743=ORIENTED_EDGE('',*,*,#4561,.T.);
#6744=ORIENTED_EDGE('',*,*,#4560,.F.);
#6745=ORIENTED_EDGE('',*,*,#4946,.T.);
#6746=ORIENTED_EDGE('',*,*,#4520,.F.);
#6747=ORIENTED_EDGE('',*,*,#4946,.F.);
#6748=ORIENTED_EDGE('',*,*,#4554,.F.);
#6749=ORIENTED_EDGE('',*,*,#4945,.F.);
#8274=PLANE('',#9303);
#8275=PLANE('',#9307);
#8276=PLANE('',#9311);
#8277=PLANE('',#9315);
#8278=PLANE('',#9321);
#8279=PLANE('',#9324);
#8280=PLANE('',#9325);
#8281=PLANE('',#9331);
#8282=PLANE('',#9334);
#8283=PLANE('',#9337);
#8284=PLANE('',#9341);
#8285=PLANE('',#9345);
#8286=PLANE('',#9348);
#8287=PLANE('',#9351);
#8288=PLANE('',#9352);
#8289=PLANE('',#9353);
#8290=PLANE('',#9360);
#8291=PLANE('',#9368);
#8292=PLANE('',#9374);
#8293=PLANE('',#9375);
#8294=PLANE('',#9384);
#8295=PLANE('',#9385);
#8296=PLANE('',#9386);
#8297=PLANE('',#9387);
#8298=PLANE('',#9389);
#8299=PLANE('',#9392);
#8300=PLANE('',#9394);
#8301=PLANE('',#9396);
#8302=PLANE('',#9397);
#8303=PLANE('',#9398);
#8304=PLANE('',#9399);
#8305=PLANE('',#9400);
#8306=PLANE('',#9401);
#8307=PLANE('',#9402);
#8308=PLANE('',#9403);
#8309=PLANE('',#9404);
#8310=PLANE('',#9405);
#8311=PLANE('',#9406);
#8312=PLANE('',#9407);
#8313=PLANE('',#9408);
#8314=PLANE('',#9409);
#8315=PLANE('',#9410);
#8316=PLANE('',#9411);
#8317=PLANE('',#9412);
#8318=PLANE('',#9413);
#8319=PLANE('',#9414);
#8320=PLANE('',#9415);
#8321=PLANE('',#9416);
#8322=PLANE('',#9417);
#8323=PLANE('',#9418);
#8324=PLANE('',#9419);
#8325=PLANE('',#9420);
#8326=PLANE('',#9421);
#8327=PLANE('',#9422);
#8328=PLANE('',#9423);
#8329=PLANE('',#9424);
#8330=PLANE('',#9425);
#8331=PLANE('',#9426);
#8332=PLANE('',#9427);
#8333=PLANE('',#9428);
#8334=PLANE('',#9429);
#8335=PLANE('',#9430);
#8336=PLANE('',#9431);
#8337=PLANE('',#9432);
#8338=PLANE('',#9433);
#8339=PLANE('',#9434);
#8340=PLANE('',#9435);
#8341=PLANE('',#9436);
#8342=PLANE('',#9437);
#8343=PLANE('',#9438);
#8344=PLANE('',#9439);
#8345=PLANE('',#9440);
#8346=PLANE('',#9441);
#8347=PLANE('',#9442);
#8348=PLANE('',#9443);
#8349=PLANE('',#9444);
#8350=PLANE('',#9445);
#8351=PLANE('',#9446);
#8352=PLANE('',#9447);
#8353=PLANE('',#9448);
#8354=PLANE('',#9449);
#8355=PLANE('',#9450);
#8356=PLANE('',#9451);
#8357=PLANE('',#9452);
#8358=PLANE('',#9453);
#8359=PLANE('',#9454);
#8360=PLANE('',#9455);
#8361=PLANE('',#9456);
#8362=PLANE('',#9457);
#8363=PLANE('',#9458);
#8364=PLANE('',#9459);
#8365=PLANE('',#9460);
#8366=PLANE('',#9461);
#8367=PLANE('',#9469);
#8602=ADVANCED_FACE('',(#881),#8274,.T.);
#8603=ADVANCED_FACE('',(#882),#368,.T.);
#8604=ADVANCED_FACE('',(#883),#8275,.T.);
#8605=ADVANCED_FACE('',(#884),#369,.T.);
#8606=ADVANCED_FACE('',(#885),#8276,.T.);
#8607=ADVANCED_FACE('',(#886),#370,.T.);
#8608=ADVANCED_FACE('',(#887),#8277,.T.);
#8609=ADVANCED_FACE('',(#888),#371,.T.);
#8610=ADVANCED_FACE('',(#889),#499,.T.);
#8611=ADVANCED_FACE('',(#890),#8278,.T.);
#8612=ADVANCED_FACE('',(#891),#500,.T.);
#8613=ADVANCED_FACE('',(#892),#8279,.T.);
#8614=ADVANCED_FACE('',(#893,#585,#586,#587,#588,#589),#8280,.T.);
#8615=ADVANCED_FACE('',(#894),#8281,.T.);
#8616=ADVANCED_FACE('',(#895),#372,.T.);
#8617=ADVANCED_FACE('',(#896),#8282,.T.);
#8618=ADVANCED_FACE('',(#897),#373,.T.);
#8619=ADVANCED_FACE('',(#898),#8283,.T.);
#8620=ADVANCED_FACE('',(#899),#374,.T.);
#8621=ADVANCED_FACE('',(#900),#8284,.T.);
#8622=ADVANCED_FACE('',(#901),#375,.T.);
#8623=ADVANCED_FACE('',(#902),#8285,.T.);
#8624=ADVANCED_FACE('',(#903),#376,.T.);
#8625=ADVANCED_FACE('',(#904),#8286,.T.);
#8626=ADVANCED_FACE('',(#905),#377,.T.);
#8627=ADVANCED_FACE('',(#906),#8287,.T.);
#8628=ADVANCED_FACE('',(#907),#8288,.T.);
#8629=ADVANCED_FACE('',(#908),#143,.F.);
#8630=ADVANCED_FACE('',(#909),#8289,.T.);
#8631=ADVANCED_FACE('',(#910),#378,.F.);
#8632=ADVANCED_FACE('',(#911),#379,.T.);
#8633=ADVANCED_FACE('',(#912),#8290,.T.);
#8634=ADVANCED_FACE('',(#913),#380,.F.);
#8635=ADVANCED_FACE('',(#914),#381,.F.);
#8636=ADVANCED_FACE('',(#915),#382,.T.);
#8637=ADVANCED_FACE('',(#916),#8291,.T.);
#8638=ADVANCED_FACE('',(#917),#383,.F.);
#8639=ADVANCED_FACE('',(#918),#384,.F.);
#8640=ADVANCED_FACE('',(#919),#8292,.T.);
#8641=ADVANCED_FACE('',(#920,#590,#591,#592,#593,#594,#595,#596,#597),#8293,
 .T.);
#8642=ADVANCED_FACE('',(#921),#385,.F.);
#8643=ADVANCED_FACE('',(#922),#386,.F.);
#8644=ADVANCED_FACE('',(#923),#387,.F.);
#8645=ADVANCED_FACE('',(#924),#8294,.T.);
#8646=ADVANCED_FACE('',(#925),#8295,.F.);
#8647=ADVANCED_FACE('',(#926),#8296,.F.);
#8648=ADVANCED_FACE('',(#927),#8297,.T.);
#8649=ADVANCED_FACE('',(#928),#388,.T.);
#8650=ADVANCED_FACE('',(#929),#8298,.T.);
#8651=ADVANCED_FACE('',(#930),#389,.T.);
#8652=ADVANCED_FACE('',(#931),#8299,.T.);
#8653=ADVANCED_FACE('',(#932),#390,.T.);
#8654=ADVANCED_FACE('',(#933),#8300,.T.);
#8655=ADVANCED_FACE('',(#934),#391,.T.);
#8656=ADVANCED_FACE('',(#935),#8301,.F.);
#8657=ADVANCED_FACE('',(#936),#8302,.F.);
#8658=ADVANCED_FACE('',(#937),#8303,.T.);
#8659=ADVANCED_FACE('',(#938),#8304,.F.);
#8660=ADVANCED_FACE('',(#939),#8305,.F.);
#8661=ADVANCED_FACE('',(#940),#8306,.F.);
#8662=ADVANCED_FACE('',(#941),#8307,.F.);
#8663=ADVANCED_FACE('',(#942),#8308,.F.);
#8664=ADVANCED_FACE('',(#943),#8309,.F.);
#8665=ADVANCED_FACE('',(#944),#8310,.F.);
#8666=ADVANCED_FACE('',(#945),#8311,.F.);
#8667=ADVANCED_FACE('',(#946),#8312,.F.);
#8668=ADVANCED_FACE('',(#947),#8313,.F.);
#8669=ADVANCED_FACE('',(#948),#8314,.F.);
#8670=ADVANCED_FACE('',(#949),#8315,.F.);
#8671=ADVANCED_FACE('',(#950),#8316,.F.);
#8672=ADVANCED_FACE('',(#951),#8317,.F.);
#8673=ADVANCED_FACE('',(#952),#8318,.F.);
#8674=ADVANCED_FACE('',(#953),#8319,.F.);
#8675=ADVANCED_FACE('',(#954),#144,.F.);
#8676=ADVANCED_FACE('',(#955),#145,.F.);
#8677=ADVANCED_FACE('',(#956),#146,.F.);
#8678=ADVANCED_FACE('',(#957),#147,.F.);
#8679=ADVANCED_FACE('',(#958),#148,.F.);
#8680=ADVANCED_FACE('',(#959),#149,.F.);
#8681=ADVANCED_FACE('',(#960),#8320,.F.);
#8682=ADVANCED_FACE('',(#961),#8321,.F.);
#8683=ADVANCED_FACE('',(#962),#8322,.F.);
#8684=ADVANCED_FACE('',(#963),#8323,.F.);
#8685=ADVANCED_FACE('',(#964),#8324,.F.);
#8686=ADVANCED_FACE('',(#965),#8325,.F.);
#8687=ADVANCED_FACE('',(#966),#8326,.F.);
#8688=ADVANCED_FACE('',(#967),#8327,.F.);
#8689=ADVANCED_FACE('',(#968),#8328,.F.);
#8690=ADVANCED_FACE('',(#969),#8329,.F.);
#8691=ADVANCED_FACE('',(#970),#8330,.F.);
#8692=ADVANCED_FACE('',(#971),#8331,.F.);
#8693=ADVANCED_FACE('',(#972),#8332,.F.);
#8694=ADVANCED_FACE('',(#973),#8333,.F.);
#8695=ADVANCED_FACE('',(#974),#8334,.F.);
#8696=ADVANCED_FACE('',(#975),#8335,.F.);
#8697=ADVANCED_FACE('',(#976),#8336,.F.);
#8698=ADVANCED_FACE('',(#977),#8337,.F.);
#8699=ADVANCED_FACE('',(#978),#8338,.F.);
#8700=ADVANCED_FACE('',(#979),#8339,.F.);
#8701=ADVANCED_FACE('',(#980),#8340,.F.);
#8702=ADVANCED_FACE('',(#981),#8341,.F.);
#8703=ADVANCED_FACE('',(#982),#150,.F.);
#8704=ADVANCED_FACE('',(#983),#151,.F.);
#8705=ADVANCED_FACE('',(#984),#152,.F.);
#8706=ADVANCED_FACE('',(#985),#153,.F.);
#8707=ADVANCED_FACE('',(#986),#154,.F.);
#8708=ADVANCED_FACE('',(#987),#155,.F.);
#8709=ADVANCED_FACE('',(#988),#156,.F.);
#8710=ADVANCED_FACE('',(#989),#157,.F.);
#8711=ADVANCED_FACE('',(#990),#158,.F.);
#8712=ADVANCED_FACE('',(#991),#159,.F.);
#8713=ADVANCED_FACE('',(#992),#160,.F.);
#8714=ADVANCED_FACE('',(#993),#8342,.T.);
#8715=ADVANCED_FACE('',(#994),#8343,.F.);
#8716=ADVANCED_FACE('',(#995),#8344,.F.);
#8717=ADVANCED_FACE('',(#996),#8345,.F.);
#8718=ADVANCED_FACE('',(#997),#8346,.F.);
#8719=ADVANCED_FACE('',(#998),#8347,.F.);
#8720=ADVANCED_FACE('',(#999),#8348,.F.);
#8721=ADVANCED_FACE('',(#1000),#8349,.F.);
#8722=ADVANCED_FACE('',(#1001),#8350,.F.);
#8723=ADVANCED_FACE('',(#1002),#8351,.F.);
#8724=ADVANCED_FACE('',(#1003),#8352,.F.);
#8725=ADVANCED_FACE('',(#1004),#8353,.F.);
#8726=ADVANCED_FACE('',(#1005),#161,.F.);
#8727=ADVANCED_FACE('',(#1006),#162,.F.);
#8728=ADVANCED_FACE('',(#1007),#163,.F.);
#8729=ADVANCED_FACE('',(#1008),#164,.F.);
#8730=ADVANCED_FACE('',(#1009),#165,.F.);
#8731=ADVANCED_FACE('',(#1010),#166,.F.);
#8732=ADVANCED_FACE('',(#1011),#167,.F.);
#8733=ADVANCED_FACE('',(#1012),#168,.F.);
#8734=ADVANCED_FACE('',(#1013),#169,.F.);
#8735=ADVANCED_FACE('',(#1014),#170,.F.);
#8736=ADVANCED_FACE('',(#1015),#171,.F.);
#8737=ADVANCED_FACE('',(#1016),#8354,.T.);
#8738=ADVANCED_FACE('',(#1017),#8355,.F.);
#8739=ADVANCED_FACE('',(#1018),#8356,.F.);
#8740=ADVANCED_FACE('',(#1019),#8357,.F.);
#8741=ADVANCED_FACE('',(#1020),#8358,.F.);
#8742=ADVANCED_FACE('',(#1021),#8359,.F.);
#8743=ADVANCED_FACE('',(#1022),#8360,.F.);
#8744=ADVANCED_FACE('',(#1023),#8361,.F.);
#8745=ADVANCED_FACE('',(#1024),#8362,.F.);
#8746=ADVANCED_FACE('',(#1025),#8363,.F.);
#8747=ADVANCED_FACE('',(#1026),#8364,.F.);
#8748=ADVANCED_FACE('',(#1027),#8365,.F.);
#8749=ADVANCED_FACE('',(#1028),#172,.F.);
#8750=ADVANCED_FACE('',(#1029),#173,.F.);
#8751=ADVANCED_FACE('',(#1030),#174,.F.);
#8752=ADVANCED_FACE('',(#1031),#175,.F.);
#8753=ADVANCED_FACE('',(#1032),#176,.F.);
#8754=ADVANCED_FACE('',(#1033),#177,.F.);
#8755=ADVANCED_FACE('',(#1034),#178,.F.);
#8756=ADVANCED_FACE('',(#1035),#179,.F.);
#8757=ADVANCED_FACE('',(#1036),#180,.F.);
#8758=ADVANCED_FACE('',(#1037),#181,.F.);
#8759=ADVANCED_FACE('',(#1038),#182,.F.);
#8760=ADVANCED_FACE('',(#1039),#8366,.T.);
#8761=ADVANCED_FACE('',(#1040),#501,.F.);
#8762=ADVANCED_FACE('',(#1041),#502,.F.);
#8763=ADVANCED_FACE('',(#1042),#503,.F.);
#8764=ADVANCED_FACE('',(#1043),#504,.F.);
#8765=ADVANCED_FACE('',(#1044),#505,.F.);
#8766=ADVANCED_FACE('',(#1045),#506,.T.);
#8767=ADVANCED_FACE('',(#1046),#507,.T.);
#8768=ADVANCED_FACE('',(#1047),#8367,.T.);
#9087=CLOSED_SHELL('',(#8602,#8603,#8604,#8605,#8606,#8607,#8608,#8609,
#8610,#8611,#8612,#8613,#8614,#8615,#8616,#8617,#8618,#8619,#8620,#8621,
#8622,#8623,#8624,#8625,#8626,#8627,#8628,#8629,#8630,#8631,#8632,#8633,
#8634,#8635,#8636,#8637,#8638,#8639,#8640,#8641,#8642,#8643,#8644,#8645,
#8646,#8647,#8648,#8649,#8650,#8651,#8652,#8653,#8654,#8655,#8656,#8657,
#8658,#8659,#8660,#8661,#8662,#8663,#8664,#8665,#8666,#8667,#8668,#8669,
#8670,#8671,#8672,#8673,#8674,#8675,#8676,#8677,#8678,#8679,#8680,#8681,
#8682,#8683,#8684,#8685,#8686,#8687,#8688,#8689,#8690,#8691,#8692,#8693,
#8694,#8695,#8696,#8697,#8698,#8699,#8700,#8701,#8702,#8703,#8704,#8705,
#8706,#8707,#8708,#8709,#8710,#8711,#8712,#8713,#8714,#8715,#8716,#8717,
#8718,#8719,#8720,#8721,#8722,#8723,#8724,#8725,#8726,#8727,#8728,#8729,
#8730,#8731,#8732,#8733,#8734,#8735,#8736,#8737,#8738,#8739,#8740,#8741,
#8742,#8743,#8744,#8745,#8746,#8747,#8748,#8749,#8750,#8751,#8752,#8753,
#8754,#8755,#8756,#8757,#8758,#8759,#8760,#8761,#8762,#8763,#8764,#8765,
#8766,#8767,#8768));
#9302=AXIS2_PLACEMENT_3D('',#12440,#10153,#10154);
#9303=AXIS2_PLACEMENT_3D('',#12441,#10155,#10156);
#9304=AXIS2_PLACEMENT_3D('',#12450,#10161,#10162);
#9305=AXIS2_PLACEMENT_3D('',#12452,#10163,#10164);
#9306=AXIS2_PLACEMENT_3D('',#12455,#10166,#10167);
#9307=AXIS2_PLACEMENT_3D('',#12456,#10168,#10169);
#9308=AXIS2_PLACEMENT_3D('',#12462,#10173,#10174);
#9309=AXIS2_PLACEMENT_3D('',#12464,#10175,#10176);
#9310=AXIS2_PLACEMENT_3D('',#12467,#10178,#10179);
#9311=AXIS2_PLACEMENT_3D('',#12468,#10180,#10181);
#9312=AXIS2_PLACEMENT_3D('',#12474,#10185,#10186);
#9313=AXIS2_PLACEMENT_3D('',#12476,#10187,#10188);
#9314=AXIS2_PLACEMENT_3D('',#12479,#10190,#10191);
#9315=AXIS2_PLACEMENT_3D('',#12480,#10192,#10193);
#9316=AXIS2_PLACEMENT_3D('',#12486,#10197,#10198);
#9317=AXIS2_PLACEMENT_3D('',#12487,#10199,#10200);
#9318=AXIS2_PLACEMENT_3D('',#12488,#10201,#10202);
#9319=AXIS2_PLACEMENT_3D('',#12489,#10203,#10204);
#9320=AXIS2_PLACEMENT_3D('',#12493,#10206,#10207);
#9321=AXIS2_PLACEMENT_3D('',#12495,#10209,#10210);
#9322=AXIS2_PLACEMENT_3D('',#12499,#10213,#10214);
#9323=AXIS2_PLACEMENT_3D('',#12502,#10216,#10217);
#9324=AXIS2_PLACEMENT_3D('',#12503,#10218,#10219);
#9325=AXIS2_PLACEMENT_3D('',#12507,#10222,#10223);
#9326=AXIS2_PLACEMENT_3D('',#12509,#10224,#10225);
#9327=AXIS2_PLACEMENT_3D('',#12511,#10226,#10227);
#9328=AXIS2_PLACEMENT_3D('',#12513,#10228,#10229);
#9329=AXIS2_PLACEMENT_3D('',#12515,#10230,#10231);
#9330=AXIS2_PLACEMENT_3D('',#12517,#10232,#10233);
#9331=AXIS2_PLACEMENT_3D('',#12518,#10234,#10235);
#9332=AXIS2_PLACEMENT_3D('',#12526,#10240,#10241);
#9333=AXIS2_PLACEMENT_3D('',#12529,#10243,#10244);
#9334=AXIS2_PLACEMENT_3D('',#12530,#10245,#10246);
#9335=AXIS2_PLACEMENT_3D('',#12534,#10249,#10250);
#9336=AXIS2_PLACEMENT_3D('',#12537,#10252,#10253);
#9337=AXIS2_PLACEMENT_3D('',#12538,#10254,#10255);
#9338=AXIS2_PLACEMENT_3D('',#12542,#10258,#10259);
#9339=AXIS2_PLACEMENT_3D('',#12546,#10261,#10262);
#9340=AXIS2_PLACEMENT_3D('',#12547,#10263,#10264);
#9341=AXIS2_PLACEMENT_3D('',#12548,#10265,#10266);
#9342=AXIS2_PLACEMENT_3D('',#12568,#10272,#10273);
#9343=AXIS2_PLACEMENT_3D('',#12569,#10274,#10275);
#9344=AXIS2_PLACEMENT_3D('',#12570,#10276,#10277);
#9345=AXIS2_PLACEMENT_3D('',#12571,#10278,#10279);
#9346=AXIS2_PLACEMENT_3D('',#12573,#10281,#10282);
#9347=AXIS2_PLACEMENT_3D('',#12577,#10284,#10285);
#9348=AXIS2_PLACEMENT_3D('',#12579,#10287,#10288);
#9349=AXIS2_PLACEMENT_3D('',#12583,#10291,#10292);
#9350=AXIS2_PLACEMENT_3D('',#12586,#10294,#10295);
#9351=AXIS2_PLACEMENT_3D('',#12587,#10296,#10297);
#9352=AXIS2_PLACEMENT_3D('',#12623,#10308,#10309);
#9353=AXIS2_PLACEMENT_3D('',#12674,#10312,#10313);
#9354=AXIS2_PLACEMENT_3D('',#12687,#10315,#10316);
#9355=AXIS2_PLACEMENT_3D('',#12689,#10317,#10318);
#9356=AXIS2_PLACEMENT_3D('',#12693,#10320,#10321);
#9357=AXIS2_PLACEMENT_3D('',#12713,#10322,#10323);
#9358=AXIS2_PLACEMENT_3D('',#12714,#10324,#10325);
#9359=AXIS2_PLACEMENT_3D('',#12717,#10327,#10328);
#9360=AXIS2_PLACEMENT_3D('',#12719,#10330,#10331);
#9361=AXIS2_PLACEMENT_3D('',#12727,#10336,#10337);
#9362=AXIS2_PLACEMENT_3D('',#12730,#10339,#10340);
#9363=AXIS2_PLACEMENT_3D('',#12731,#10341,#10342);
#9364=AXIS2_PLACEMENT_3D('',#12733,#10343,#10344);
#9365=AXIS2_PLACEMENT_3D('',#12737,#10346,#10347);
#9366=AXIS2_PLACEMENT_3D('',#12757,#10348,#10349);
#9367=AXIS2_PLACEMENT_3D('',#12758,#10350,#10351);
#9368=AXIS2_PLACEMENT_3D('',#12761,#10354,#10355);
#9369=AXIS2_PLACEMENT_3D('',#12769,#10358,#10359);
#9370=AXIS2_PLACEMENT_3D('',#12772,#10361,#10362);
#9371=AXIS2_PLACEMENT_3D('',#12773,#10363,#10364);
#9372=AXIS2_PLACEMENT_3D('',#12775,#10365,#10366);
#9373=AXIS2_PLACEMENT_3D('',#12783,#10368,#10369);
#9374=AXIS2_PLACEMENT_3D('',#12802,#10370,#10371);
#9375=AXIS2_PLACEMENT_3D('',#12807,#10375,#10376);
#9376=AXIS2_PLACEMENT_3D('',#12810,#10378,#10379);
#9377=AXIS2_PLACEMENT_3D('',#13013,#10426,#10427);
#9378=AXIS2_PLACEMENT_3D('',#13078,#10438,#10439);
#9379=AXIS2_PLACEMENT_3D('',#13081,#10441,#10442);
#9380=AXIS2_PLACEMENT_3D('',#13082,#10443,#10444);
#9381=AXIS2_PLACEMENT_3D('',#13084,#10445,#10446);
#9382=AXIS2_PLACEMENT_3D('',#13104,#10448,#10449);
#9383=AXIS2_PLACEMENT_3D('',#13107,#10451,#10452);
#9384=AXIS2_PLACEMENT_3D('',#13108,#10453,#10454);
#9385=AXIS2_PLACEMENT_3D('',#13115,#10459,#10460);
#9386=AXIS2_PLACEMENT_3D('',#13119,#10463,#10464);
#9387=AXIS2_PLACEMENT_3D('',#13123,#10467,#10468);
#9388=AXIS2_PLACEMENT_3D('',#13124,#10469,#10470);
#9389=AXIS2_PLACEMENT_3D('',#13126,#10472,#10473);
#9390=AXIS2_PLACEMENT_3D('',#13130,#10476,#10477);
#9391=AXIS2_PLACEMENT_3D('',#13131,#10478,#10479);
#9392=AXIS2_PLACEMENT_3D('',#13132,#10480,#10481);
#9393=AXIS2_PLACEMENT_3D('',#13134,#10483,#10484);
#9394=AXIS2_PLACEMENT_3D('',#13136,#10486,#10487);
#9395=AXIS2_PLACEMENT_3D('',#13138,#10489,#10490);
#9396=AXIS2_PLACEMENT_3D('',#13139,#10491,#10492);
#9397=AXIS2_PLACEMENT_3D('',#13143,#10495,#10496);
#9398=AXIS2_PLACEMENT_3D('',#13147,#10499,#10500);
#9399=AXIS2_PLACEMENT_3D('',#13171,#10501,#10502);
#9400=AXIS2_PLACEMENT_3D('',#13175,#10505,#10506);
#9401=AXIS2_PLACEMENT_3D('',#13179,#10509,#10510);
#9402=AXIS2_PLACEMENT_3D('',#13183,#10513,#10514);
#9403=AXIS2_PLACEMENT_3D('',#13187,#10517,#10518);
#9404=AXIS2_PLACEMENT_3D('',#13191,#10521,#10522);
#9405=AXIS2_PLACEMENT_3D('',#13195,#10525,#10526);
#9406=AXIS2_PLACEMENT_3D('',#13197,#10528,#10529);
#9407=AXIS2_PLACEMENT_3D('',#13198,#10530,#10531);
#9408=AXIS2_PLACEMENT_3D('',#13202,#10534,#10535);
#9409=AXIS2_PLACEMENT_3D('',#13206,#10538,#10539);
#9410=AXIS2_PLACEMENT_3D('',#13210,#10542,#10543);
#9411=AXIS2_PLACEMENT_3D('',#13214,#10546,#10547);
#9412=AXIS2_PLACEMENT_3D('',#13218,#10550,#10551);
#9413=AXIS2_PLACEMENT_3D('',#13222,#10554,#10555);
#9414=AXIS2_PLACEMENT_3D('',#13224,#10557,#10558);
#9415=AXIS2_PLACEMENT_3D('',#13274,#10564,#10565);
#9416=AXIS2_PLACEMENT_3D('',#13280,#10569,#10570);
#9417=AXIS2_PLACEMENT_3D('',#13284,#10573,#10574);
#9418=AXIS2_PLACEMENT_3D('',#13288,#10577,#10578);
#9419=AXIS2_PLACEMENT_3D('',#13292,#10581,#10582);
#9420=AXIS2_PLACEMENT_3D('',#13296,#10585,#10586);
#9421=AXIS2_PLACEMENT_3D('',#13300,#10589,#10590);
#9422=AXIS2_PLACEMENT_3D('',#13304,#10593,#10594);
#9423=AXIS2_PLACEMENT_3D('',#13308,#10597,#10598);
#9424=AXIS2_PLACEMENT_3D('',#13312,#10601,#10602);
#9425=AXIS2_PLACEMENT_3D('',#13314,#10604,#10605);
#9426=AXIS2_PLACEMENT_3D('',#13315,#10606,#10607);
#9427=AXIS2_PLACEMENT_3D('',#13321,#10611,#10612);
#9428=AXIS2_PLACEMENT_3D('',#13325,#10615,#10616);
#9429=AXIS2_PLACEMENT_3D('',#13329,#10619,#10620);
#9430=AXIS2_PLACEMENT_3D('',#13333,#10623,#10624);
#9431=AXIS2_PLACEMENT_3D('',#13337,#10627,#10628);
#9432=AXIS2_PLACEMENT_3D('',#13341,#10631,#10632);
#9433=AXIS2_PLACEMENT_3D('',#13345,#10635,#10636);
#9434=AXIS2_PLACEMENT_3D('',#13349,#10639,#10640);
#9435=AXIS2_PLACEMENT_3D('',#13353,#10643,#10644);
#9436=AXIS2_PLACEMENT_3D('',#13355,#10646,#10647);
#9437=AXIS2_PLACEMENT_3D('',#13477,#10659,#10660);
#9438=AXIS2_PLACEMENT_3D('',#13478,#10661,#10662);
#9439=AXIS2_PLACEMENT_3D('',#13484,#10666,#10667);
#9440=AXIS2_PLACEMENT_3D('',#13488,#10670,#10671);
#9441=AXIS2_PLACEMENT_3D('',#13492,#10674,#10675);
#9442=AXIS2_PLACEMENT_3D('',#13496,#10678,#10679);
#9443=AXIS2_PLACEMENT_3D('',#13500,#10682,#10683);
#9444=AXIS2_PLACEMENT_3D('',#13504,#10686,#10687);
#9445=AXIS2_PLACEMENT_3D('',#13508,#10690,#10691);
#9446=AXIS2_PLACEMENT_3D('',#13512,#10694,#10695);
#9447=AXIS2_PLACEMENT_3D('',#13516,#10698,#10699);
#9448=AXIS2_PLACEMENT_3D('',#13518,#10701,#10702);
#9449=AXIS2_PLACEMENT_3D('',#13640,#10714,#10715);
#9450=AXIS2_PLACEMENT_3D('',#13641,#10716,#10717);
#9451=AXIS2_PLACEMENT_3D('',#13647,#10721,#10722);
#9452=AXIS2_PLACEMENT_3D('',#13651,#10725,#10726);
#9453=AXIS2_PLACEMENT_3D('',#13655,#10729,#10730);
#9454=AXIS2_PLACEMENT_3D('',#13659,#10733,#10734);
#9455=AXIS2_PLACEMENT_3D('',#13663,#10737,#10738);
#9456=AXIS2_PLACEMENT_3D('',#13667,#10741,#10742);
#9457=AXIS2_PLACEMENT_3D('',#13671,#10745,#10746);
#9458=AXIS2_PLACEMENT_3D('',#13675,#10749,#10750);
#9459=AXIS2_PLACEMENT_3D('',#13679,#10753,#10754);
#9460=AXIS2_PLACEMENT_3D('',#13681,#10756,#10757);
#9461=AXIS2_PLACEMENT_3D('',#13803,#10769,#10770);
#9462=AXIS2_PLACEMENT_3D('',#13804,#10771,#10772);
#9463=AXIS2_PLACEMENT_3D('',#13806,#10774,#10775);
#9464=AXIS2_PLACEMENT_3D('',#13808,#10777,#10778);
#9465=AXIS2_PLACEMENT_3D('',#13810,#10780,#10781);
#9466=AXIS2_PLACEMENT_3D('',#13812,#10783,#10784);
#9467=AXIS2_PLACEMENT_3D('',#13814,#10786,#10787);
#9468=AXIS2_PLACEMENT_3D('',#13816,#10789,#10790);
#9469=AXIS2_PLACEMENT_3D('',#13818,#10792,#10793);
#10153=DIRECTION('axis',(0.,0.,1.));
#10154=DIRECTION('refdir',(1.,0.,0.));
#10155=DIRECTION('center_axis',(0.707106781186548,0.707106781186547,0.));
#10156=DIRECTION('ref_axis',(0.,0.,-1.));
#10157=DIRECTION('',(0.707106781186547,-0.707106781186548,0.));
#10158=DIRECTION('',(0.,0.,-1.));
#10159=DIRECTION('',(-0.707106781186547,0.707106781186548,0.));
#10160=DIRECTION('',(0.,0.,1.));
#10161=DIRECTION('center_axis',(-1.,0.,0.));
#10162=DIRECTION('ref_axis',(0.,0.707106781186548,0.707106781186548));
#10163=DIRECTION('center_axis',(1.,0.,0.));
#10164=DIRECTION('ref_axis',(0.,0.707106781186548,0.707106781186548));
#10165=DIRECTION('',(0.707106781186555,0.,-0.70710678118654));
#10166=DIRECTION('center_axis',(-1.,0.,0.));
#10167=DIRECTION('ref_axis',(0.,0.707106781186548,0.707106781186548));
#10168=DIRECTION('center_axis',(0.70710678118654,0.,0.707106781186555));
#10169=DIRECTION('ref_axis',(0.707106781186555,0.,-0.70710678118654));
#10170=DIRECTION('',(0.707106781186555,0.,-0.70710678118654));
#10171=DIRECTION('',(0.,1.,0.));
#10172=DIRECTION('',(0.,-1.,0.));
#10173=DIRECTION('center_axis',(-1.,0.,0.));
#10174=DIRECTION('ref_axis',(0.,-0.707106781186548,0.707106781186548));
#10175=DIRECTION('center_axis',(1.,0.,0.));
#10176=DIRECTION('ref_axis',(0.,-0.707106781186548,0.707106781186548));
#10177=DIRECTION('',(0.707106781186539,0.707106781186556,0.));
#10178=DIRECTION('center_axis',(-1.,0.,0.));
#10179=DIRECTION('ref_axis',(0.,-0.707106781186548,0.707106781186548));
#10180=DIRECTION('center_axis',(0.707106781186548,-0.707106781186547,0.));
#10181=DIRECTION('ref_axis',(0.,0.,-1.));
#10182=DIRECTION('',(0.707106781186547,0.707106781186548,0.));
#10183=DIRECTION('',(0.,0.,1.));
#10184=DIRECTION('',(0.,0.,-1.));
#10185=DIRECTION('center_axis',(-1.,0.,0.));
#10186=DIRECTION('ref_axis',(0.,-0.707106781186547,-0.707106781186547));
#10187=DIRECTION('center_axis',(1.,0.,0.));
#10188=DIRECTION('ref_axis',(0.,-0.707106781186548,-0.707106781186548));
#10189=DIRECTION('',(0.707106781186539,0.,0.707106781186556));
#10190=DIRECTION('center_axis',(-1.,0.,0.));
#10191=DIRECTION('ref_axis',(0.,-0.707106781186547,-0.707106781186547));
#10192=DIRECTION('center_axis',(0.707106781186548,0.,-0.707106781186547));
#10193=DIRECTION('ref_axis',(-0.707106781186547,0.,-0.707106781186548));
#10194=DIRECTION('',(0.707106781186547,0.,0.707106781186548));
#10195=DIRECTION('',(0.,-1.,0.));
#10196=DIRECTION('',(0.,1.,0.));
#10197=DIRECTION('center_axis',(-1.,0.,0.));
#10198=DIRECTION('ref_axis',(0.,0.707106781186548,-0.707106781186547));
#10199=DIRECTION('center_axis',(1.,0.,0.));
#10200=DIRECTION('ref_axis',(0.,0.707106781186548,-0.707106781186547));
#10201=DIRECTION('center_axis',(-1.,0.,0.));
#10202=DIRECTION('ref_axis',(0.,0.707106781186548,-0.707106781186547));
#10203=DIRECTION('center_axis',(-1.,0.,0.));
#10204=DIRECTION('ref_axis',(0.,-0.707106781186548,0.707106781186548));
#10205=DIRECTION('',(-1.,0.,0.));
#10206=DIRECTION('center_axis',(-1.,0.,0.));
#10207=DIRECTION('ref_axis',(0.,-0.707106781186548,0.707106781186548));
#10208=DIRECTION('',(1.,0.,0.));
#10209=DIRECTION('center_axis',(0.,0.,1.));
#10210=DIRECTION('ref_axis',(0.,1.,0.));
#10211=DIRECTION('',(1.,0.,0.));
#10212=DIRECTION('',(0.,1.,0.));
#10213=DIRECTION('center_axis',(-1.,0.,0.));
#10214=DIRECTION('ref_axis',(0.,0.707106781186548,0.707106781186548));
#10215=DIRECTION('',(-1.,0.,0.));
#10216=DIRECTION('center_axis',(-1.,0.,0.));
#10217=DIRECTION('ref_axis',(0.,0.707106781186548,0.707106781186548));
#10218=DIRECTION('center_axis',(0.,1.,0.));
#10219=DIRECTION('ref_axis',(0.,0.,-1.));
#10220=DIRECTION('',(1.,0.,0.));
#10221=DIRECTION('',(0.,0.,-1.));
#10222=DIRECTION('center_axis',(1.,0.,0.));
#10223=DIRECTION('ref_axis',(0.,0.,-1.));
#10224=DIRECTION('center_axis',(-1.,0.,0.));
#10225=DIRECTION('ref_axis',(0.,0.,-1.));
#10226=DIRECTION('center_axis',(-1.,0.,0.));
#10227=DIRECTION('ref_axis',(0.,0.,-1.));
#10228=DIRECTION('center_axis',(-1.,0.,0.));
#10229=DIRECTION('ref_axis',(0.,0.,-1.));
#10230=DIRECTION('center_axis',(-1.,0.,0.));
#10231=DIRECTION('ref_axis',(0.,0.,-1.));
#10232=DIRECTION('center_axis',(-1.,0.,0.));
#10233=DIRECTION('ref_axis',(0.,0.,-1.));
#10234=DIRECTION('center_axis',(-0.382683432365091,-0.923879532511286,0.));
#10235=DIRECTION('ref_axis',(0.,0.,-1.));
#10236=DIRECTION('',(-0.923879532511286,0.382683432365092,0.));
#10237=DIRECTION('',(0.,0.,-1.));
#10238=DIRECTION('',(0.923879532511286,-0.382683432365091,0.));
#10239=DIRECTION('',(0.,0.,1.));
#10240=DIRECTION('center_axis',(1.,0.,0.));
#10241=DIRECTION('ref_axis',(0.,-0.707106781186547,0.707106781186548));
#10242=DIRECTION('',(-0.923879532511289,0.,-0.382683432365085));
#10243=DIRECTION('center_axis',(1.,0.,0.));
#10244=DIRECTION('ref_axis',(0.,-0.707106781186547,0.707106781186548));
#10245=DIRECTION('center_axis',(-0.382683432365079,0.,0.923879532511291));
#10246=DIRECTION('ref_axis',(0.923879532511291,0.,0.382683432365079));
#10247=DIRECTION('',(-0.92387953251129,0.,-0.382683432365081));
#10248=DIRECTION('',(0.,-1.,0.));
#10249=DIRECTION('center_axis',(1.,0.,0.));
#10250=DIRECTION('ref_axis',(0.,0.707106781186547,0.707106781186548));
#10251=DIRECTION('',(-0.923879532511288,-0.382683432365088,0.));
#10252=DIRECTION('center_axis',(1.,0.,0.));
#10253=DIRECTION('ref_axis',(0.,0.707106781186547,0.707106781186548));
#10254=DIRECTION('center_axis',(-0.382683432365091,0.923879532511286,0.));
#10255=DIRECTION('ref_axis',(0.,0.,1.));
#10256=DIRECTION('',(-0.923879532511286,-0.382683432365091,0.));
#10257=DIRECTION('',(0.,0.,1.));
#10258=DIRECTION('center_axis',(1.,0.,0.));
#10259=DIRECTION('ref_axis',(0.,0.707106781186548,-0.707106781186547));
#10260=DIRECTION('',(-0.92387953251129,0.,0.382683432365082));
#10261=DIRECTION('center_axis',(1.,0.,0.));
#10262=DIRECTION('ref_axis',(0.,0.707106781186548,-0.707106781186547));
#10263=DIRECTION('center_axis',(-1.,0.,0.));
#10264=DIRECTION('ref_axis',(0.,0.707106781186548,-0.707106781186547));
#10265=DIRECTION('center_axis',(-0.382683432365091,0.,-0.923879532511286));
#10266=DIRECTION('ref_axis',(-0.923879532511286,0.,0.382683432365091));
#10267=DIRECTION('',(0.,1.,0.));
#10268=DIRECTION('',(0.,-1.,0.));
#10269=DIRECTION('',(-0.923879532511286,0.,0.382683432365092));
#10270=DIRECTION('',(0.,1.,0.));
#10271=DIRECTION('',(-6.49886142244849E-16,1.,2.69191654116148E-16));
#10272=DIRECTION('center_axis',(1.,0.,0.));
#10273=DIRECTION('ref_axis',(0.,-0.707106781186547,-0.707106781186547));
#10274=DIRECTION('center_axis',(1.,0.,0.));
#10275=DIRECTION('ref_axis',(0.,-0.707106781186548,-0.707106781186548));
#10276=DIRECTION('center_axis',(-1.,0.,0.));
#10277=DIRECTION('ref_axis',(0.,-0.707106781186548,-0.707106781186548));
#10278=DIRECTION('center_axis',(0.,-1.,0.));
#10279=DIRECTION('ref_axis',(0.,0.,1.));
#10280=DIRECTION('',(-1.,0.,0.));
#10281=DIRECTION('center_axis',(1.,0.,0.));
#10282=DIRECTION('ref_axis',(0.,0.707106781186547,0.707106781186547));
#10283=DIRECTION('',(0.707106781186549,0.707106781186546,0.));
#10284=DIRECTION('center_axis',(-1.,0.,0.));
#10285=DIRECTION('ref_axis',(0.,0.707106781186547,0.707106781186548));
#10286=DIRECTION('',(0.707106781186542,0.,0.707106781186553));
#10287=DIRECTION('center_axis',(-0.707106781186546,0.707106781186549,0.));
#10288=DIRECTION('ref_axis',(0.,0.,1.));
#10289=DIRECTION('',(0.707106781186549,0.707106781186546,6.28036983473511E-15));
#10290=DIRECTION('',(0.,0.,-1.));
#10291=DIRECTION('center_axis',(1.,0.,0.));
#10292=DIRECTION('ref_axis',(0.,0.707106781186548,-0.707106781186547));
#10293=DIRECTION('',(0.707106781186549,0.,-0.707106781186546));
#10294=DIRECTION('center_axis',(-1.,0.,0.));
#10295=DIRECTION('ref_axis',(0.,0.707106781186548,-0.707106781186547));
#10296=DIRECTION('center_axis',(-0.707106781186546,0.,-0.707106781186549));
#10297=DIRECTION('ref_axis',(-0.707106781186549,0.,0.707106781186546));
#10298=DIRECTION('',(0.707106781186542,0.,-0.707106781186553));
#10299=DIRECTION('',(0.,-1.,0.));
#10300=DIRECTION('',(0.707106781186549,0.,-0.707106781186546));
#10301=DIRECTION('',(0.,1.,0.));
#10302=DIRECTION('',(-0.707106781186549,0.,0.707106781186546));
#10303=DIRECTION('',(0.,-1.,0.));
#10304=DIRECTION('',(0.707106781186549,9.8130778667736E-17,-0.707106781186546));
#10305=DIRECTION('',(-1.38777878078144E-16,1.,1.38777878078144E-16));
#10306=DIRECTION('',(-0.707106781186549,-9.8130778667736E-17,0.707106781186546));
#10307=DIRECTION('',(0.,1.,0.));
#10308=DIRECTION('center_axis',(-0.707106781186546,0.,-0.707106781186549));
#10309=DIRECTION('ref_axis',(-0.707106781186549,0.,0.707106781186546));
#10310=DIRECTION('',(0.,-1.,0.));
#10311=DIRECTION('',(1.,0.,0.));
#10312=DIRECTION('center_axis',(-0.923879532511287,-4.97401319121531E-16,
-0.382683432365089));
#10313=DIRECTION('ref_axis',(-0.382683432365089,0.,0.923879532511287));
#10314=DIRECTION('',(-9.19077796360991E-16,1.,9.19077796360989E-16));
#10315=DIRECTION('center_axis',(-1.,0.,0.));
#10316=DIRECTION('ref_axis',(0.,0.,-1.));
#10317=DIRECTION('center_axis',(1.,-1.42859248789192E-15,0.));
#10318=DIRECTION('ref_axis',(0.,0.,-1.));
#10319=DIRECTION('',(-0.382683432365103,-1.13142611228769E-16,0.923879532511281));
#10320=DIRECTION('center_axis',(-1.,0.,0.));
#10321=DIRECTION('ref_axis',(0.,0.,-1.));
#10322=DIRECTION('center_axis',(-1.,0.,0.));
#10323=DIRECTION('ref_axis',(0.,0.,-1.));
#10324=DIRECTION('center_axis',(1.,0.,0.));
#10325=DIRECTION('ref_axis',(0.,-0.707106781186548,-0.707106781186548));
#10326=DIRECTION('',(0.38268343236509,0.,-0.923879532511287));
#10327=DIRECTION('center_axis',(-1.,0.,0.));
#10328=DIRECTION('ref_axis',(0.,-0.707106781186548,-0.707106781186548));
#10329=DIRECTION('',(0.382683432365099,-0.923879532511283,0.));
#10330=DIRECTION('center_axis',(-0.923879532511282,0.,-0.382683432365101));
#10331=DIRECTION('ref_axis',(-0.382683432365101,0.,0.923879532511282));
#10332=DIRECTION('',(0.,1.,0.));
#10333=DIRECTION('',(0.382683432365101,0.,-0.923879532511282));
#10334=DIRECTION('',(0.,1.,0.));
#10335=DIRECTION('',(0.382683432365101,0.,-0.923879532511282));
#10336=DIRECTION('center_axis',(-1.,0.,0.));
#10337=DIRECTION('ref_axis',(0.,0.,-1.));
#10338=DIRECTION('',(0.707106781186548,-8.65956056235493E-17,-0.707106781186547));
#10339=DIRECTION('center_axis',(1.,0.,0.));
#10340=DIRECTION('ref_axis',(0.,0.,-1.));
#10341=DIRECTION('center_axis',(-1.,0.,0.));
#10342=DIRECTION('ref_axis',(0.,0.,-1.));
#10343=DIRECTION('center_axis',(1.,-1.42859248789192E-15,0.));
#10344=DIRECTION('ref_axis',(0.,0.,-1.));
#10345=DIRECTION('',(-0.382683432365103,-1.13142611228769E-16,0.923879532511281));
#10346=DIRECTION('center_axis',(-1.,0.,0.));
#10347=DIRECTION('ref_axis',(0.,0.,-1.));
#10348=DIRECTION('center_axis',(-1.,0.,0.));
#10349=DIRECTION('ref_axis',(0.,0.,-1.));
#10350=DIRECTION('center_axis',(1.,0.,0.));
#10351=DIRECTION('ref_axis',(0.,0.707106781186548,-0.707106781186547));
#10352=DIRECTION('',(0.382683432365085,0.923879532511289,-1.2016967424393E-14));
#10353=DIRECTION('',(0.382683432365099,0.,-0.923879532511283));
#10354=DIRECTION('center_axis',(-0.923879532511282,0.382683432365101,0.));
#10355=DIRECTION('ref_axis',(0.,0.,1.));
#10356=DIRECTION('',(0.,0.,1.));
#10357=DIRECTION('',(0.382683432365099,0.923879532511283,0.));
#10358=DIRECTION('center_axis',(-1.,0.,0.));
#10359=DIRECTION('ref_axis',(0.,0.,-1.));
#10360=DIRECTION('',(0.707106781186548,-8.65956056235493E-17,-0.707106781186547));
#10361=DIRECTION('center_axis',(1.,0.,0.));
#10362=DIRECTION('ref_axis',(0.,0.,-1.));
#10363=DIRECTION('center_axis',(-1.,0.,0.));
#10364=DIRECTION('ref_axis',(0.,0.,-1.));
#10365=DIRECTION('center_axis',(1.,-1.60716654887841E-15,0.));
#10366=DIRECTION('ref_axis',(0.,0.,-1.));
#10367=DIRECTION('',(-0.382683432365116,-1.13142611228769E-16,0.923879532511276));
#10368=DIRECTION('center_axis',(-1.,0.,0.));
#10369=DIRECTION('ref_axis',(0.,0.,-1.));
#10370=DIRECTION('center_axis',(-0.923879532511282,-0.382683432365101,0.));
#10371=DIRECTION('ref_axis',(0.,0.,1.));
#10372=DIRECTION('',(0.,0.,1.));
#10373=DIRECTION('',(0.3826834323651,-0.923879532511283,0.));
#10374=DIRECTION('',(0.,0.,-1.));
#10375=DIRECTION('center_axis',(-1.,0.,0.));
#10376=DIRECTION('ref_axis',(0.,0.,1.));
#10377=DIRECTION('',(0.,-1.,0.));
#10378=DIRECTION('center_axis',(-1.,0.,0.));
#10379=DIRECTION('ref_axis',(0.,0.,-1.));
#10380=DIRECTION('',(0.,1.,0.));
#10381=DIRECTION('',(0.,-1.69953884180861E-32,1.));
#10382=DIRECTION('',(0.,-1.,0.));
#10383=DIRECTION('',(0.,1.69953884180861E-32,-1.));
#10384=DIRECTION('',(0.,1.,0.));
#10385=DIRECTION('',(0.,1.69953884180861E-32,-1.));
#10386=DIRECTION('',(0.,-1.,0.));
#10387=DIRECTION('',(0.,1.69953884180861E-32,-1.));
#10388=DIRECTION('',(0.,1.,0.));
#10389=DIRECTION('',(0.,0.,1.));
#10390=DIRECTION('',(0.,-1.,0.));
#10391=DIRECTION('',(0.,0.,-1.));
#10392=DIRECTION('',(0.,1.,0.));
#10393=DIRECTION('',(0.,0.,-1.));
#10394=DIRECTION('',(0.,-1.,0.));
#10395=DIRECTION('',(0.,0.,-1.));
#10396=DIRECTION('',(0.,1.,0.));
#10397=DIRECTION('',(0.,0.,-1.));
#10398=DIRECTION('',(0.,1.,0.));
#10399=DIRECTION('',(0.,0.,1.));
#10400=DIRECTION('',(0.,-1.,0.));
#10401=DIRECTION('',(0.,0.,-1.));
#10402=DIRECTION('',(0.,1.,0.));
#10403=DIRECTION('',(0.,0.,-1.));
#10404=DIRECTION('',(0.,-1.,0.));
#10405=DIRECTION('',(0.,0.,-1.));
#10406=DIRECTION('',(0.,1.,0.));
#10407=DIRECTION('',(0.,1.69953884180861E-32,-1.));
#10408=DIRECTION('',(0.,1.,0.));
#10409=DIRECTION('',(0.,-1.69953884180861E-32,1.));
#10410=DIRECTION('',(0.,-1.,0.));
#10411=DIRECTION('',(0.,1.69953884180861E-32,-1.));
#10412=DIRECTION('',(0.,1.,0.));
#10413=DIRECTION('',(0.,1.69953884180861E-32,-1.));
#10414=DIRECTION('',(0.,-1.,0.));
#10415=DIRECTION('',(0.,1.69953884180861E-32,-1.));
#10416=DIRECTION('',(0.,0.55569909667333,0.831383493916282));
#10417=DIRECTION('',(0.,0.,-1.));
#10418=DIRECTION('',(0.,1.,0.));
#10419=DIRECTION('',(0.,0.,1.));
#10420=DIRECTION('',(0.,-1.,0.));
#10421=DIRECTION('',(0.,-0.556032657337733,-0.831160444182673));
#10422=DIRECTION('',(0.,0.,1.));
#10423=DIRECTION('',(0.,-1.,0.));
#10424=DIRECTION('',(0.,0.,-1.));
#10425=DIRECTION('',(0.,1.,0.));
#10426=DIRECTION('center_axis',(1.,0.,0.));
#10427=DIRECTION('ref_axis',(0.,0.,-1.));
#10428=DIRECTION('',(0.,0.55569909667333,0.831383493916282));
#10429=DIRECTION('',(0.,0.,-1.));
#10430=DIRECTION('',(0.,1.,0.));
#10431=DIRECTION('',(0.,0.,1.));
#10432=DIRECTION('',(0.,-1.,0.));
#10433=DIRECTION('',(0.,-0.556032657337733,-0.831160444182673));
#10434=DIRECTION('',(0.,0.,1.));
#10435=DIRECTION('',(0.,-1.,0.));
#10436=DIRECTION('',(0.,0.,-1.));
#10437=DIRECTION('',(0.,1.,0.));
#10438=DIRECTION('center_axis',(-1.,0.,0.));
#10439=DIRECTION('ref_axis',(0.,0.,-1.));
#10440=DIRECTION('',(0.707106781186547,-8.65956056235494E-17,-0.707106781186548));
#10441=DIRECTION('center_axis',(1.,0.,0.));
#10442=DIRECTION('ref_axis',(0.,0.,-1.));
#10443=DIRECTION('center_axis',(-1.,0.,0.));
#10444=DIRECTION('ref_axis',(0.,0.,-1.));
#10445=DIRECTION('center_axis',(1.,-1.60716654887841E-15,0.));
#10446=DIRECTION('ref_axis',(0.,0.,-1.));
#10447=DIRECTION('',(-0.382683432365116,-1.13142611228769E-16,0.923879532511276));
#10448=DIRECTION('center_axis',(-1.,0.,0.));
#10449=DIRECTION('ref_axis',(0.,0.,-1.));
#10450=DIRECTION('',(0.707106781186547,-8.65956056235494E-17,-0.707106781186548));
#10451=DIRECTION('center_axis',(1.,0.,0.));
#10452=DIRECTION('ref_axis',(0.,0.,-1.));
#10453=DIRECTION('center_axis',(-0.923879532511282,0.,-0.382683432365101));
#10454=DIRECTION('ref_axis',(-0.382683432365101,0.,0.923879532511282));
#10455=DIRECTION('',(-0.382683432365101,0.,0.923879532511282));
#10456=DIRECTION('',(0.382683432365101,5.31079947192899E-17,-0.923879532511282));
#10457=DIRECTION('',(0.,1.,0.));
#10458=DIRECTION('',(0.382683432365101,5.31079947192899E-17,-0.923879532511282));
#10459=DIRECTION('center_axis',(1.38777878078144E-16,-1.,-1.69953884180861E-32));
#10460=DIRECTION('ref_axis',(-1.22464679914735E-16,0.,-1.));
#10461=DIRECTION('',(1.,1.38777878078144E-16,0.));
#10462=DIRECTION('',(-1.22464679914735E-16,0.,-1.));
#10463=DIRECTION('center_axis',(0.,0.,-1.));
#10464=DIRECTION('ref_axis',(-1.22464679914735E-16,1.,0.));
#10465=DIRECTION('',(1.,1.38777878078144E-16,0.));
#10466=DIRECTION('',(-1.22464679914735E-16,1.,0.));
#10467=DIRECTION('center_axis',(-0.923879532511282,0.,-0.382683432365101));
#10468=DIRECTION('ref_axis',(-0.382683432365101,0.,0.923879532511282));
#10469=DIRECTION('center_axis',(1.,0.,0.));
#10470=DIRECTION('ref_axis',(0.,0.707106781186547,0.707106781186548));
#10471=DIRECTION('',(0.382683432365096,-1.20169674243929E-14,0.923879532511284));
#10472=DIRECTION('center_axis',(-0.923879532511287,0.,0.38268343236509));
#10473=DIRECTION('ref_axis',(0.38268343236509,0.,0.923879532511286));
#10474=DIRECTION('',(0.382683432365112,0.,0.923879532511278));
#10475=DIRECTION('',(0.,1.,0.));
#10476=DIRECTION('center_axis',(1.,0.,0.));
#10477=DIRECTION('ref_axis',(7.9970871068614E-17,-0.707106781186547,0.707106781186548));
#10478=DIRECTION('center_axis',(-1.,-2.15587857746042E-16,0.));
#10479=DIRECTION('ref_axis',(1.52443636153707E-16,-0.707106781186547,0.707106781186548));
#10480=DIRECTION('center_axis',(-0.707106781186546,0.,0.707106781186549));
#10481=DIRECTION('ref_axis',(0.707106781186549,0.,0.707106781186546));
#10482=DIRECTION('',(-0.707106781186542,0.,-0.707106781186553));
#10483=DIRECTION('center_axis',(1.,0.,0.));
#10484=DIRECTION('ref_axis',(0.,-0.707106781186547,0.707106781186547));
#10485=DIRECTION('',(0.707106781186542,-0.707106781186553,0.));
#10486=DIRECTION('center_axis',(-0.707106781186546,-0.707106781186549,0.));
#10487=DIRECTION('ref_axis',(0.,0.,1.));
#10488=DIRECTION('',(0.707106781186549,-0.707106781186546,0.));
#10489=DIRECTION('center_axis',(1.,0.,0.));
#10490=DIRECTION('ref_axis',(0.,-0.707106781186547,-0.707106781186547));
#10491=DIRECTION('center_axis',(0.,-1.,0.));
#10492=DIRECTION('ref_axis',(-1.22464679914735E-16,0.,-1.));
#10493=DIRECTION('',(1.,0.,0.));
#10494=DIRECTION('',(-1.22464679914735E-16,0.,-1.));
#10495=DIRECTION('center_axis',(0.,0.,-1.));
#10496=DIRECTION('ref_axis',(-1.22464679914735E-16,1.,0.));
#10497=DIRECTION('',(1.,0.,0.));
#10498=DIRECTION('',(-1.22464679914735E-16,1.,0.));
#10499=DIRECTION('center_axis',(-1.,-9.19077796360991E-16,-2.78913508712442E-16));
#10500=DIRECTION('ref_axis',(-2.78913508712442E-16,0.,1.));
#10501=DIRECTION('center_axis',(0.,-1.,0.));
#10502=DIRECTION('ref_axis',(-1.22464679914735E-16,0.,-1.));
#10503=DIRECTION('',(1.,0.,0.));
#10504=DIRECTION('',(-1.22464679914735E-16,0.,-1.));
#10505=DIRECTION('center_axis',(0.,0.,1.));
#10506=DIRECTION('ref_axis',(1.22464679914735E-16,-1.,0.));
#10507=DIRECTION('',(1.,0.,0.));
#10508=DIRECTION('',(1.22464679914735E-16,-1.,0.));
#10509=DIRECTION('center_axis',(0.,-1.,0.));
#10510=DIRECTION('ref_axis',(-1.22464679914735E-16,0.,-1.));
#10511=DIRECTION('',(1.,0.,0.));
#10512=DIRECTION('',(-1.22464679914735E-16,0.,-1.));
#10513=DIRECTION('center_axis',(0.,0.,-1.));
#10514=DIRECTION('ref_axis',(-1.22464679914735E-16,1.,0.));
#10515=DIRECTION('',(1.,0.,0.));
#10516=DIRECTION('',(-1.22464679914735E-16,1.,0.));
#10517=DIRECTION('center_axis',(0.,-1.,0.));
#10518=DIRECTION('ref_axis',(-1.22464679914735E-16,0.,-1.));
#10519=DIRECTION('',(1.,0.,0.));
#10520=DIRECTION('',(-1.22464679914735E-16,0.,-1.));
#10521=DIRECTION('center_axis',(0.,0.,1.));
#10522=DIRECTION('ref_axis',(1.22464679914735E-16,-1.,0.));
#10523=DIRECTION('',(1.,0.,0.));
#10524=DIRECTION('',(1.22464679914735E-16,-1.,0.));
#10525=DIRECTION('center_axis',(0.,1.,0.));
#10526=DIRECTION('ref_axis',(1.22464679914735E-16,0.,1.));
#10527=DIRECTION('',(1.22464679914735E-16,0.,1.));
#10528=DIRECTION('center_axis',(1.,0.,0.));
#10529=DIRECTION('ref_axis',(0.,0.,-1.));
#10530=DIRECTION('center_axis',(1.38777878078144E-16,-1.,-1.69953884180861E-32));
#10531=DIRECTION('ref_axis',(-1.22464679914735E-16,0.,-1.));
#10532=DIRECTION('',(1.,1.38777878078144E-16,0.));
#10533=DIRECTION('',(-1.22464679914735E-16,0.,-1.));
#10534=DIRECTION('center_axis',(0.,0.,1.));
#10535=DIRECTION('ref_axis',(1.22464679914735E-16,-1.,0.));
#10536=DIRECTION('',(1.,1.38777878078144E-16,0.));
#10537=DIRECTION('',(1.22464679914735E-16,-1.,0.));
#10538=DIRECTION('center_axis',(1.38777878078144E-16,-1.,-1.69953884180861E-32));
#10539=DIRECTION('ref_axis',(-1.22464679914735E-16,0.,-1.));
#10540=DIRECTION('',(1.,1.38777878078144E-16,0.));
#10541=DIRECTION('',(-1.22464679914735E-16,0.,-1.));
#10542=DIRECTION('center_axis',(0.,0.,-1.));
#10543=DIRECTION('ref_axis',(-1.22464679914735E-16,1.,0.));
#10544=DIRECTION('',(1.,1.38777878078144E-16,0.));
#10545=DIRECTION('',(-1.22464679914735E-16,1.,0.));
#10546=DIRECTION('center_axis',(1.38777878078144E-16,-1.,-1.69953884180861E-32));
#10547=DIRECTION('ref_axis',(-1.22464679914735E-16,0.,-1.));
#10548=DIRECTION('',(1.,1.38777878078144E-16,0.));
#10549=DIRECTION('',(-1.22464679914735E-16,0.,-1.));
#10550=DIRECTION('center_axis',(0.,0.,1.));
#10551=DIRECTION('ref_axis',(1.22464679914735E-16,-1.,0.));
#10552=DIRECTION('',(1.,1.38777878078144E-16,0.));
#10553=DIRECTION('',(1.22464679914735E-16,-1.,0.));
#10554=DIRECTION('center_axis',(-1.38777878078144E-16,1.,1.69953884180861E-32));
#10555=DIRECTION('ref_axis',(1.22464679914735E-16,0.,1.));
#10556=DIRECTION('',(1.22464679914735E-16,0.,1.));
#10557=DIRECTION('center_axis',(1.,1.38777878078144E-16,0.));
#10558=DIRECTION('ref_axis',(0.,0.,-1.));
#10559=DIRECTION('',(1.,0.,0.));
#10560=DIRECTION('',(1.,0.,0.));
#10561=DIRECTION('',(1.,0.,0.));
#10562=DIRECTION('',(1.,0.,0.));
#10563=DIRECTION('',(1.,0.,0.));
#10564=DIRECTION('center_axis',(0.,0.,-1.));
#10565=DIRECTION('ref_axis',(-1.22464679914735E-16,1.,0.));
#10566=DIRECTION('',(1.,0.,0.));
#10567=DIRECTION('',(-1.22464679914735E-16,1.,0.));
#10568=DIRECTION('',(1.,0.,0.));
#10569=DIRECTION('center_axis',(0.,-1.,0.));
#10570=DIRECTION('ref_axis',(-1.22464679914735E-16,0.,-1.));
#10571=DIRECTION('',(1.,0.,0.));
#10572=DIRECTION('',(-1.22464679914735E-16,0.,-1.));
#10573=DIRECTION('center_axis',(0.,0.,1.));
#10574=DIRECTION('ref_axis',(1.22464679914735E-16,-1.,0.));
#10575=DIRECTION('',(1.,0.,0.));
#10576=DIRECTION('',(1.22464679914735E-16,-1.,0.));
#10577=DIRECTION('center_axis',(0.,-1.,0.));
#10578=DIRECTION('ref_axis',(-1.22464679914735E-16,0.,-1.));
#10579=DIRECTION('',(1.,0.,0.));
#10580=DIRECTION('',(-1.22464679914735E-16,0.,-1.));
#10581=DIRECTION('center_axis',(0.,0.,-1.));
#10582=DIRECTION('ref_axis',(-1.22464679914735E-16,1.,0.));
#10583=DIRECTION('',(1.,0.,0.));
#10584=DIRECTION('',(-1.22464679914735E-16,1.,0.));
#10585=DIRECTION('center_axis',(0.,-1.,0.));
#10586=DIRECTION('ref_axis',(-1.22464679914735E-16,0.,-1.));
#10587=DIRECTION('',(1.,0.,0.));
#10588=DIRECTION('',(-1.22464679914735E-16,0.,-1.));
#10589=DIRECTION('center_axis',(0.,0.,1.));
#10590=DIRECTION('ref_axis',(1.22464679914735E-16,-1.,0.));
#10591=DIRECTION('',(1.,0.,0.));
#10592=DIRECTION('',(1.22464679914735E-16,-1.,0.));
#10593=DIRECTION('center_axis',(0.,1.,0.));
#10594=DIRECTION('ref_axis',(1.22464679914735E-16,0.,1.));
#10595=DIRECTION('',(1.,0.,0.));
#10596=DIRECTION('',(1.22464679914735E-16,0.,1.));
#10597=DIRECTION('center_axis',(0.,0.,-1.));
#10598=DIRECTION('ref_axis',(-1.22464679914735E-16,1.,0.));
#10599=DIRECTION('',(1.,0.,0.));
#10600=DIRECTION('',(-1.22464679914735E-16,1.,0.));
#10601=DIRECTION('center_axis',(0.,-1.,0.));
#10602=DIRECTION('ref_axis',(-1.22464679914735E-16,0.,-1.));
#10603=DIRECTION('',(-1.22464679914735E-16,0.,-1.));
#10604=DIRECTION('center_axis',(1.,0.,0.));
#10605=DIRECTION('ref_axis',(0.,0.,-1.));
#10606=DIRECTION('center_axis',(0.,0.,-1.));
#10607=DIRECTION('ref_axis',(-1.22464679914735E-16,1.,0.));
#10608=DIRECTION('',(1.,1.38777878078144E-16,0.));
#10609=DIRECTION('',(-1.22464679914735E-16,1.,0.));
#10610=DIRECTION('',(1.,1.38777878078144E-16,0.));
#10611=DIRECTION('center_axis',(1.38777878078144E-16,-1.,-1.69953884180861E-32));
#10612=DIRECTION('ref_axis',(-1.22464679914735E-16,0.,-1.));
#10613=DIRECTION('',(1.,1.38777878078144E-16,0.));
#10614=DIRECTION('',(-1.22464679914735E-16,0.,-1.));
#10615=DIRECTION('center_axis',(0.,0.,1.));
#10616=DIRECTION('ref_axis',(1.22464679914735E-16,-1.,0.));
#10617=DIRECTION('',(1.,1.38777878078144E-16,0.));
#10618=DIRECTION('',(1.22464679914735E-16,-1.,0.));
#10619=DIRECTION('center_axis',(1.38777878078144E-16,-1.,-1.69953884180861E-32));
#10620=DIRECTION('ref_axis',(-1.22464679914735E-16,0.,-1.));
#10621=DIRECTION('',(1.,1.38777878078144E-16,0.));
#10622=DIRECTION('',(-1.22464679914735E-16,0.,-1.));
#10623=DIRECTION('center_axis',(0.,0.,-1.));
#10624=DIRECTION('ref_axis',(-1.22464679914735E-16,1.,0.));
#10625=DIRECTION('',(1.,1.38777878078144E-16,0.));
#10626=DIRECTION('',(-1.22464679914735E-16,1.,0.));
#10627=DIRECTION('center_axis',(1.38777878078144E-16,-1.,-1.69953884180861E-32));
#10628=DIRECTION('ref_axis',(-1.22464679914735E-16,0.,-1.));
#10629=DIRECTION('',(1.,1.38777878078144E-16,0.));
#10630=DIRECTION('',(-1.22464679914735E-16,0.,-1.));
#10631=DIRECTION('center_axis',(0.,0.,1.));
#10632=DIRECTION('ref_axis',(1.22464679914735E-16,-1.,0.));
#10633=DIRECTION('',(1.,1.38777878078144E-16,0.));
#10634=DIRECTION('',(1.22464679914735E-16,-1.,0.));
#10635=DIRECTION('center_axis',(-1.38777878078144E-16,1.,1.69953884180861E-32));
#10636=DIRECTION('ref_axis',(1.22464679914735E-16,0.,1.));
#10637=DIRECTION('',(1.,1.38777878078144E-16,0.));
#10638=DIRECTION('',(1.22464679914735E-16,0.,1.));
#10639=DIRECTION('center_axis',(0.,0.,-1.));
#10640=DIRECTION('ref_axis',(-1.22464679914735E-16,1.,0.));
#10641=DIRECTION('',(1.,1.38777878078144E-16,0.));
#10642=DIRECTION('',(-1.22464679914735E-16,1.,0.));
#10643=DIRECTION('center_axis',(1.38777878078144E-16,-1.,-1.69953884180861E-32));
#10644=DIRECTION('ref_axis',(-1.22464679914735E-16,0.,-1.));
#10645=DIRECTION('',(-1.22464679914735E-16,0.,-1.));
#10646=DIRECTION('center_axis',(1.,1.38777878078144E-16,0.));
#10647=DIRECTION('ref_axis',(0.,0.,-1.));
#10648=DIRECTION('',(1.,0.,0.));
#10649=DIRECTION('',(1.,0.,0.));
#10650=DIRECTION('',(1.,0.,0.));
#10651=DIRECTION('',(1.,0.,0.));
#10652=DIRECTION('',(1.,0.,0.));
#10653=DIRECTION('',(1.,0.,0.));
#10654=DIRECTION('',(1.,0.,0.));
#10655=DIRECTION('',(1.,0.,0.));
#10656=DIRECTION('',(1.,0.,0.));
#10657=DIRECTION('',(1.,0.,0.));
#10658=DIRECTION('',(1.,0.,0.));
#10659=DIRECTION('center_axis',(-1.,-9.19077796360991E-16,-2.78913508712442E-16));
#10660=DIRECTION('ref_axis',(-2.78913508712442E-16,0.,1.));
#10661=DIRECTION('center_axis',(0.,0.831383493916282,-0.55569909667333));
#10662=DIRECTION('ref_axis',(3.37616014658449E-17,0.55569909667333,0.831383493916282));
#10663=DIRECTION('',(1.,0.,0.));
#10664=DIRECTION('',(3.37616014658449E-17,0.55569909667333,0.831383493916282));
#10665=DIRECTION('',(1.,0.,0.));
#10666=DIRECTION('center_axis',(0.,0.,-1.));
#10667=DIRECTION('ref_axis',(-1.22464679914735E-16,1.,0.));
#10668=DIRECTION('',(1.,0.,0.));
#10669=DIRECTION('',(-1.22464679914735E-16,1.,0.));
#10670=DIRECTION('center_axis',(0.,-1.,0.));
#10671=DIRECTION('ref_axis',(-1.22464679914735E-16,0.,-1.));
#10672=DIRECTION('',(1.,0.,0.));
#10673=DIRECTION('',(-1.22464679914735E-16,0.,-1.));
#10674=DIRECTION('center_axis',(0.,0.,1.));
#10675=DIRECTION('ref_axis',(1.22464679914735E-16,-1.,0.));
#10676=DIRECTION('',(1.,0.,0.));
#10677=DIRECTION('',(1.22464679914735E-16,-1.,0.));
#10678=DIRECTION('center_axis',(0.,1.,0.));
#10679=DIRECTION('ref_axis',(1.22464679914735E-16,0.,1.));
#10680=DIRECTION('',(1.,0.,0.));
#10681=DIRECTION('',(1.22464679914735E-16,0.,1.));
#10682=DIRECTION('center_axis',(0.,-0.831160444182673,0.556032657337733));
#10683=DIRECTION('ref_axis',(-3.36934363516151E-17,-0.556032657337733,-0.831160444182673));
#10684=DIRECTION('',(1.,0.,0.));
#10685=DIRECTION('',(-3.36934363516151E-17,-0.556032657337733,-0.831160444182673));
#10686=DIRECTION('center_axis',(0.,0.,1.));
#10687=DIRECTION('ref_axis',(1.22464679914735E-16,-1.,0.));
#10688=DIRECTION('',(1.,0.,0.));
#10689=DIRECTION('',(1.22464679914735E-16,-1.,0.));
#10690=DIRECTION('center_axis',(0.,1.,0.));
#10691=DIRECTION('ref_axis',(1.22464679914735E-16,0.,1.));
#10692=DIRECTION('',(1.,0.,0.));
#10693=DIRECTION('',(1.22464679914735E-16,0.,1.));
#10694=DIRECTION('center_axis',(0.,0.,-1.));
#10695=DIRECTION('ref_axis',(-1.22464679914735E-16,1.,0.));
#10696=DIRECTION('',(1.,0.,0.));
#10697=DIRECTION('',(-1.22464679914735E-16,1.,0.));
#10698=DIRECTION('center_axis',(0.,-1.,0.));
#10699=DIRECTION('ref_axis',(-1.22464679914735E-16,0.,-1.));
#10700=DIRECTION('',(-1.22464679914735E-16,0.,-1.));
#10701=DIRECTION('center_axis',(1.,0.,0.));
#10702=DIRECTION('ref_axis',(0.,0.,-1.));
#10703=DIRECTION('',(1.,0.,0.));
#10704=DIRECTION('',(1.,0.,0.));
#10705=DIRECTION('',(1.,0.,0.));
#10706=DIRECTION('',(1.,0.,0.));
#10707=DIRECTION('',(1.,0.,0.));
#10708=DIRECTION('',(1.,0.,0.));
#10709=DIRECTION('',(1.,0.,0.));
#10710=DIRECTION('',(1.,0.,0.));
#10711=DIRECTION('',(1.,0.,0.));
#10712=DIRECTION('',(1.,0.,0.));
#10713=DIRECTION('',(1.,0.,0.));
#10714=DIRECTION('center_axis',(-1.,-9.1907723979186E-16,-2.78913274147473E-16));
#10715=DIRECTION('ref_axis',(-2.78913274147473E-16,0.,1.));
#10716=DIRECTION('center_axis',(0.,0.831383493916282,-0.55569909667333));
#10717=DIRECTION('ref_axis',(3.37616014658449E-17,0.55569909667333,0.831383493916282));
#10718=DIRECTION('',(1.,0.,0.));
#10719=DIRECTION('',(3.37616014658449E-17,0.55569909667333,0.831383493916282));
#10720=DIRECTION('',(1.,0.,0.));
#10721=DIRECTION('center_axis',(0.,0.,-1.));
#10722=DIRECTION('ref_axis',(-1.22464679914735E-16,1.,0.));
#10723=DIRECTION('',(1.,0.,0.));
#10724=DIRECTION('',(-1.22464679914735E-16,1.,0.));
#10725=DIRECTION('center_axis',(0.,-1.,0.));
#10726=DIRECTION('ref_axis',(-1.22464679914735E-16,0.,-1.));
#10727=DIRECTION('',(1.,0.,0.));
#10728=DIRECTION('',(-1.22464679914735E-16,0.,-1.));
#10729=DIRECTION('center_axis',(0.,0.,1.));
#10730=DIRECTION('ref_axis',(1.22464679914735E-16,-1.,0.));
#10731=DIRECTION('',(1.,0.,0.));
#10732=DIRECTION('',(1.22464679914735E-16,-1.,0.));
#10733=DIRECTION('center_axis',(0.,1.,0.));
#10734=DIRECTION('ref_axis',(1.22464679914735E-16,0.,1.));
#10735=DIRECTION('',(1.,0.,0.));
#10736=DIRECTION('',(1.22464679914735E-16,0.,1.));
#10737=DIRECTION('center_axis',(0.,-0.831160444182673,0.556032657337733));
#10738=DIRECTION('ref_axis',(-3.36934363516151E-17,-0.556032657337733,-0.831160444182673));
#10739=DIRECTION('',(1.,0.,0.));
#10740=DIRECTION('',(-3.36934363516151E-17,-0.556032657337733,-0.831160444182673));
#10741=DIRECTION('center_axis',(0.,0.,1.));
#10742=DIRECTION('ref_axis',(1.22464679914735E-16,-1.,0.));
#10743=DIRECTION('',(1.,0.,0.));
#10744=DIRECTION('',(1.22464679914735E-16,-1.,0.));
#10745=DIRECTION('center_axis',(0.,1.,0.));
#10746=DIRECTION('ref_axis',(1.22464679914735E-16,0.,1.));
#10747=DIRECTION('',(1.,0.,0.));
#10748=DIRECTION('',(1.22464679914735E-16,0.,1.));
#10749=DIRECTION('center_axis',(0.,0.,-1.));
#10750=DIRECTION('ref_axis',(-1.22464679914735E-16,1.,0.));
#10751=DIRECTION('',(1.,0.,0.));
#10752=DIRECTION('',(-1.22464679914735E-16,1.,0.));
#10753=DIRECTION('center_axis',(0.,-1.,0.));
#10754=DIRECTION('ref_axis',(-1.22464679914735E-16,0.,-1.));
#10755=DIRECTION('',(-1.22464679914735E-16,0.,-1.));
#10756=DIRECTION('center_axis',(1.,0.,0.));
#10757=DIRECTION('ref_axis',(0.,0.,-1.));
#10758=DIRECTION('',(1.,0.,0.));
#10759=DIRECTION('',(1.,0.,0.));
#10760=DIRECTION('',(1.,0.,0.));
#10761=DIRECTION('',(1.,0.,0.));
#10762=DIRECTION('',(1.,0.,0.));
#10763=DIRECTION('',(1.,0.,0.));
#10764=DIRECTION('',(1.,0.,0.));
#10765=DIRECTION('',(1.,0.,0.));
#10766=DIRECTION('',(1.,0.,0.));
#10767=DIRECTION('',(1.,0.,0.));
#10768=DIRECTION('',(1.,0.,0.));
#10769=DIRECTION('center_axis',(-1.,-9.19077239791859E-16,-2.78913274147473E-16));
#10770=DIRECTION('ref_axis',(-2.78913274147473E-16,0.,1.));
#10771=DIRECTION('center_axis',(1.,0.,0.));
#10772=DIRECTION('ref_axis',(0.,0.,-1.));
#10773=DIRECTION('',(1.,0.,0.));
#10774=DIRECTION('center_axis',(1.,0.,0.));
#10775=DIRECTION('ref_axis',(0.,0.,-1.));
#10776=DIRECTION('',(1.,0.,0.));
#10777=DIRECTION('center_axis',(1.,0.,0.));
#10778=DIRECTION('ref_axis',(0.,0.,-1.));
#10779=DIRECTION('',(1.,0.,0.));
#10780=DIRECTION('center_axis',(1.,0.,0.));
#10781=DIRECTION('ref_axis',(0.,0.,-1.));
#10782=DIRECTION('',(1.,0.,0.));
#10783=DIRECTION('center_axis',(1.,0.,0.));
#10784=DIRECTION('ref_axis',(0.,0.,-1.));
#10785=DIRECTION('',(1.,0.,0.));
#10786=DIRECTION('center_axis',(-1.,0.,0.));
#10787=DIRECTION('ref_axis',(0.,0.707106781186548,-0.707106781186547));
#10788=DIRECTION('',(-1.,0.,0.));
#10789=DIRECTION('center_axis',(-1.,0.,0.));
#10790=DIRECTION('ref_axis',(0.,-0.707106781186548,-0.707106781186548));
#10791=DIRECTION('',(1.,0.,0.));
#10792=DIRECTION('center_axis',(0.,0.,-1.));
#10793=DIRECTION('ref_axis',(0.,-1.,0.));
#12440=CARTESIAN_POINT('',(0.,0.,0.));
#12441=CARTESIAN_POINT('Origin',(-0.1,29.,58.575));
#12442=CARTESIAN_POINT('',(-0.2,29.1,66.6));
#12443=CARTESIAN_POINT('',(0.,28.9,66.6));
#12444=CARTESIAN_POINT('',(-0.2,29.1,66.6));
#12445=CARTESIAN_POINT('',(0.,28.9,26.5));
#12446=CARTESIAN_POINT('',(0.,28.9,58.575));
#12447=CARTESIAN_POINT('',(-0.2,29.1,26.5));
#12448=CARTESIAN_POINT('',(0.,28.9,26.5));
#12449=CARTESIAN_POINT('',(-0.2,29.1,58.575));
#12450=CARTESIAN_POINT('Origin',(-0.1,25.1,66.6));
#12451=CARTESIAN_POINT('',(-0.2,25.1,70.6));
#12452=CARTESIAN_POINT('Origin',(-0.2,25.1,66.6));
#12453=CARTESIAN_POINT('',(0.,25.1,70.4));
#12454=CARTESIAN_POINT('',(-0.2,25.1,70.6));
#12455=CARTESIAN_POINT('Origin',(0.,25.1,66.6));
#12456=CARTESIAN_POINT('Origin',(-0.1,-14.55,70.5));
#12457=CARTESIAN_POINT('',(-0.2,-25.1,70.6));
#12458=CARTESIAN_POINT('',(0.,-25.1,70.4));
#12459=CARTESIAN_POINT('',(-0.2,-25.1,70.6));
#12460=CARTESIAN_POINT('',(0.,-14.55,70.4));
#12461=CARTESIAN_POINT('',(-0.2,-14.55,70.6));
#12462=CARTESIAN_POINT('Origin',(-0.1,-25.1,66.6));
#12463=CARTESIAN_POINT('',(-0.2,-29.1,66.6));
#12464=CARTESIAN_POINT('Origin',(-0.2,-25.1,66.6));
#12465=CARTESIAN_POINT('',(0.,-28.9,66.6));
#12466=CARTESIAN_POINT('',(-0.2,-29.1,66.6));
#12467=CARTESIAN_POINT('Origin',(0.,-25.1,66.6));
#12468=CARTESIAN_POINT('Origin',(-0.1,-29.,34.525));
#12469=CARTESIAN_POINT('',(-0.2,-29.1,26.5));
#12470=CARTESIAN_POINT('',(0.,-28.9,26.5));
#12471=CARTESIAN_POINT('',(-0.2,-29.1,26.5));
#12472=CARTESIAN_POINT('',(0.,-28.9,34.525));
#12473=CARTESIAN_POINT('',(-0.2,-29.1,34.525));
#12474=CARTESIAN_POINT('Origin',(-0.1,-25.1,26.5));
#12475=CARTESIAN_POINT('',(-0.2,-25.1,22.5));
#12476=CARTESIAN_POINT('Origin',(-0.2,-25.1,26.5));
#12477=CARTESIAN_POINT('',(0.,-25.1,22.7));
#12478=CARTESIAN_POINT('',(-0.2,-25.1,22.5));
#12479=CARTESIAN_POINT('Origin',(0.,-25.1,26.5));
#12480=CARTESIAN_POINT('Origin',(-0.1,14.55,22.6));
#12481=CARTESIAN_POINT('',(-0.2,25.1,22.5));
#12482=CARTESIAN_POINT('',(0.,25.1,22.7));
#12483=CARTESIAN_POINT('',(-0.2,25.1,22.5));
#12484=CARTESIAN_POINT('',(0.,14.55,22.7));
#12485=CARTESIAN_POINT('',(-0.2,14.55,22.5));
#12486=CARTESIAN_POINT('Origin',(-0.1,25.1,26.5));
#12487=CARTESIAN_POINT('Origin',(-0.2,25.1,26.5));
#12488=CARTESIAN_POINT('Origin',(0.,25.1,26.5));
#12489=CARTESIAN_POINT('Origin',(0.,-25.1,66.6));
#12490=CARTESIAN_POINT('',(-2.3,-25.1,70.6));
#12491=CARTESIAN_POINT('',(0.,-25.1,70.6));
#12492=CARTESIAN_POINT('',(-2.3,-29.1,66.6));
#12493=CARTESIAN_POINT('Origin',(-2.3,-25.1,66.6));
#12494=CARTESIAN_POINT('',(0.,-29.1,66.6));
#12495=CARTESIAN_POINT('Origin',(0.,-29.1,70.6));
#12496=CARTESIAN_POINT('',(-2.3,25.1,70.6));
#12497=CARTESIAN_POINT('',(0.,25.1,70.6));
#12498=CARTESIAN_POINT('',(-2.3,-21.825,70.6));
#12499=CARTESIAN_POINT('Origin',(0.,25.1,66.6));
#12500=CARTESIAN_POINT('',(-2.3,29.1,66.6));
#12501=CARTESIAN_POINT('',(0.,29.1,66.6));
#12502=CARTESIAN_POINT('Origin',(-2.3,25.1,66.6));
#12503=CARTESIAN_POINT('Origin',(0.,29.1,70.6));
#12504=CARTESIAN_POINT('',(-2.3,29.1,26.5));
#12505=CARTESIAN_POINT('',(0.,29.1,26.5));
#12506=CARTESIAN_POINT('',(-2.3,29.1,64.5875));
#12507=CARTESIAN_POINT('Origin',(0.,0.,46.55));
#12508=CARTESIAN_POINT('',(0.,25.,28.2));
#12509=CARTESIAN_POINT('Origin',(0.,25.,26.5));
#12510=CARTESIAN_POINT('',(0.,-25.,68.2));
#12511=CARTESIAN_POINT('Origin',(0.,-25.,66.5));
#12512=CARTESIAN_POINT('',(0.,-25.,28.2));
#12513=CARTESIAN_POINT('Origin',(0.,-25.,26.5));
#12514=CARTESIAN_POINT('',(0.,25.,68.2));
#12515=CARTESIAN_POINT('Origin',(0.,25.,66.5));
#12516=CARTESIAN_POINT('',(0.,7.9602041944578E-16,54.));
#12517=CARTESIAN_POINT('Origin',(0.,0.,47.5));
#12518=CARTESIAN_POINT('Origin',(-2.47071067811866,-29.0292893218814,28.5125));
#12519=CARTESIAN_POINT('',(-2.64142135623731,-28.9585786437627,66.6));
#12520=CARTESIAN_POINT('',(-2.3,-29.1,66.6));
#12521=CARTESIAN_POINT('',(-2.64142135623731,-28.9585786437627,26.5));
#12522=CARTESIAN_POINT('',(-2.64142135623731,-28.9585786437627,28.5125));
#12523=CARTESIAN_POINT('',(-2.3,-29.1,26.5));
#12524=CARTESIAN_POINT('',(-2.64142135623731,-28.9585786437627,26.5));
#12525=CARTESIAN_POINT('',(-2.3,-29.1,28.5125));
#12526=CARTESIAN_POINT('Origin',(-2.47071067811865,-25.1,66.6));
#12527=CARTESIAN_POINT('',(-2.6414213562373,-25.1,70.4585786437627));
#12528=CARTESIAN_POINT('',(-2.3,-25.1,70.6));
#12529=CARTESIAN_POINT('Origin',(-2.64142135623731,-25.1,66.6));
#12530=CARTESIAN_POINT('Origin',(-2.47071067811865,-21.825,70.5292893218814));
#12531=CARTESIAN_POINT('',(-2.64142135623731,25.1,70.4585786437627));
#12532=CARTESIAN_POINT('',(-2.3,25.1,70.6));
#12533=CARTESIAN_POINT('',(-2.64142135623731,-21.825,70.4585786437627));
#12534=CARTESIAN_POINT('Origin',(-2.47071067811865,25.1,66.6));
#12535=CARTESIAN_POINT('',(-2.64142135623731,28.9585786437627,66.6));
#12536=CARTESIAN_POINT('',(-2.3,29.1,66.6));
#12537=CARTESIAN_POINT('Origin',(-2.64142135623731,25.1,66.6));
#12538=CARTESIAN_POINT('Origin',(-2.47071067811866,29.0292893218814,64.5875));
#12539=CARTESIAN_POINT('',(-2.64142135623731,28.9585786437627,26.5));
#12540=CARTESIAN_POINT('',(-2.3,29.1,26.5));
#12541=CARTESIAN_POINT('',(-2.64142135623731,28.9585786437627,64.5875));
#12542=CARTESIAN_POINT('Origin',(-2.47071067811865,25.1,26.5));
#12543=CARTESIAN_POINT('',(-2.3,25.1,22.5));
#12544=CARTESIAN_POINT('',(-2.64142135623731,25.1,22.6414213562373));
#12545=CARTESIAN_POINT('',(-2.3,25.1,22.5));
#12546=CARTESIAN_POINT('Origin',(-2.64142135623731,25.1,26.5));
#12547=CARTESIAN_POINT('Origin',(-2.3,25.1,26.5));
#12548=CARTESIAN_POINT('Origin',(-2.47071067811866,21.825,22.5707106781187));
#12549=CARTESIAN_POINT('',(-2.61819805153193,4.14309288132937,22.6318019484637));
#12550=CARTESIAN_POINT('',(-2.64142135623725,4.14658995368148,22.6414213562372));
#12551=CARTESIAN_POINT('Ctrl Pts',(-2.61819805153193,4.14309288132937,22.6318019484637));
#12552=CARTESIAN_POINT('Ctrl Pts',(-2.6259378790126,4.14426860505579,22.6350078899766));
#12553=CARTESIAN_POINT('Ctrl Pts',(-2.63367898747496,4.14543428596151,22.638214362091));
#12554=CARTESIAN_POINT('Ctrl Pts',(-2.64142135623725,4.14658995368148,22.6414213562372));
#12555=CARTESIAN_POINT('',(-2.64142135623731,21.825,22.6414213562373));
#12556=CARTESIAN_POINT('',(-2.3,-25.1,22.5));
#12557=CARTESIAN_POINT('',(-2.3,21.825,22.5));
#12558=CARTESIAN_POINT('',(-2.64142135623731,-25.1,22.6414213562373));
#12559=CARTESIAN_POINT('',(-2.3,-25.1,22.5));
#12560=CARTESIAN_POINT('',(-2.64142135623721,1.29697164052348,22.6414213562372));
#12561=CARTESIAN_POINT('',(-2.64142135623731,21.825,22.6414213562373));
#12562=CARTESIAN_POINT('',(-2.61819805153393,1.30034092007739,22.631801948466));
#12563=CARTESIAN_POINT('Ctrl Pts',(-2.64142135623721,1.29697164052832,22.6414213562231));
#12564=CARTESIAN_POINT('Ctrl Pts',(-2.63367876608245,1.29808438048699,22.6382142703778));
#12565=CARTESIAN_POINT('Ctrl Pts',(-2.62593762971128,1.29920745199881,22.6350077867096));
#12566=CARTESIAN_POINT('Ctrl Pts',(-2.61819805153393,1.30034092007804,22.6318019484642));
#12567=CARTESIAN_POINT('',(-2.61819805153395,15.230763933342,22.6318019484661));
#12568=CARTESIAN_POINT('Origin',(-2.47071067811865,-25.1,26.5));
#12569=CARTESIAN_POINT('Origin',(-2.64142135623731,-25.1,26.5));
#12570=CARTESIAN_POINT('Origin',(-2.3,-25.1,26.5));
#12571=CARTESIAN_POINT('Origin',(0.,-29.1,22.5));
#12572=CARTESIAN_POINT('',(0.,-29.1,26.5));
#12573=CARTESIAN_POINT('Origin',(-2.75,25.1,66.6));
#12574=CARTESIAN_POINT('',(-2.85857864376269,28.7414213562373,66.6));
#12575=CARTESIAN_POINT('',(-3.,28.6,66.6));
#12576=CARTESIAN_POINT('',(-2.85857864376269,25.1,70.2414213562373));
#12577=CARTESIAN_POINT('Origin',(-2.85857864376269,25.1,66.6));
#12578=CARTESIAN_POINT('',(-3.,25.1,70.1));
#12579=CARTESIAN_POINT('Origin',(-2.75,28.85,58.575));
#12580=CARTESIAN_POINT('',(-2.85857864376269,28.7414213562373,26.5));
#12581=CARTESIAN_POINT('',(-3.,28.6,26.5));
#12582=CARTESIAN_POINT('',(-2.85857864376269,28.7414213562373,52.5625));
#12583=CARTESIAN_POINT('Origin',(-2.75,25.1,26.5));
#12584=CARTESIAN_POINT('',(-2.85857864376269,25.1,22.8585786437627));
#12585=CARTESIAN_POINT('',(-3.,25.1,23.));
#12586=CARTESIAN_POINT('Origin',(-2.85857864376269,25.1,26.5));
#12587=CARTESIAN_POINT('Origin',(-2.75,14.55,22.75));
#12588=CARTESIAN_POINT('',(-2.85857864376269,-25.1,22.8585786437627));
#12589=CARTESIAN_POINT('',(-3.,-25.1,23.));
#12590=CARTESIAN_POINT('',(-2.85857864376269,-2.52878561615944,22.8585786437627));
#12591=CARTESIAN_POINT('',(-2.85857864376269,7.275,22.8585786437627));
#12592=CARTESIAN_POINT('',(-2.75,-2.52878561615944,22.75));
#12593=CARTESIAN_POINT('',(-2.91343792378902,-2.52878561615944,22.913437923789));
#12594=CARTESIAN_POINT('',(-2.75,-2.10532046854496,22.75));
#12595=CARTESIAN_POINT('',(-2.75,5.68263995423913,22.75));
#12596=CARTESIAN_POINT('',(-2.85857864376269,-2.10532046854496,22.8585786437627));
#12597=CARTESIAN_POINT('',(-2.55000001788139,-2.10532046854496,22.5500000178814));
#12598=CARTESIAN_POINT('',(-2.85857864376269,0.201909989118576,22.8585786437627));
#12599=CARTESIAN_POINT('',(-2.85857864376269,7.275,22.8585786437627));
#12600=CARTESIAN_POINT('',(-2.75,0.201909989118576,22.75));
#12601=CARTESIAN_POINT('',(-2.91343792378902,0.201909989118576,22.913437923789));
#12602=CARTESIAN_POINT('',(-2.75,0.625375136733055,22.75));
#12603=CARTESIAN_POINT('',(-2.75,7.04798775687814,22.75));
#12604=CARTESIAN_POINT('',(-3.,0.625375136733055,23.));
#12605=CARTESIAN_POINT('',(-2.55000001788139,0.625375136733055,22.5500000178814));
#12606=CARTESIAN_POINT('',(-3.,1.21228337796395,23.));
#12607=CARTESIAN_POINT('',(-3.,14.55,23.));
#12608=CARTESIAN_POINT('',(-2.75,1.26319920824794,22.75));
#12609=CARTESIAN_POINT('Ctrl Pts',(-3.,1.21228337796395,23.));
#12610=CARTESIAN_POINT('Ctrl Pts',(-2.961213895248,1.21754813042459,22.961213895248));
#12611=CARTESIAN_POINT('Ctrl Pts',(-2.92250031201436,1.22395187924894,22.9225003120144));
#12612=CARTESIAN_POINT('Ctrl Pts',(-2.88391049622622,1.23157435155926,22.8839104962262));
#12613=CARTESIAN_POINT('Ctrl Pts',(-2.83908487466434,1.24042855446668,22.8390848746643));
#12614=CARTESIAN_POINT('Ctrl Pts',(-2.7944213152606,1.25092814815388,22.7944213152606));
#12615=CARTESIAN_POINT('Ctrl Pts',(-2.75,1.26319920824794,22.75));
#12616=CARTESIAN_POINT('Ctrl Pts',(-2.6414213562372,1.29697164052344,22.6414213562372));
#12617=CARTESIAN_POINT('Ctrl Pts',(-2.66759311479328,1.28789101002667,22.6675931147933));
#12618=CARTESIAN_POINT('Ctrl Pts',(-2.69302939122751,1.27976201495126,22.693031510606));
#12619=CARTESIAN_POINT('Ctrl Pts',(-2.71789496870931,1.27239069164872,22.7178960977404));
#12620=CARTESIAN_POINT('Ctrl Pts',(-2.72869989814678,1.26918760383774,22.7287005968387));
#12621=CARTESIAN_POINT('Ctrl Pts',(-2.73939706851147,1.26612818972238,22.7393970685115));
#12622=CARTESIAN_POINT('Ctrl Pts',(-2.75,1.26319920824794,22.75));
#12623=CARTESIAN_POINT('Origin',(-2.75,14.55,22.75));
#12624=CARTESIAN_POINT('',(-2.75,4.18187951621146,22.75));
#12625=CARTESIAN_POINT('Ctrl Pts',(-2.75,4.18187951621146,22.75));
#12626=CARTESIAN_POINT('Ctrl Pts',(-2.72593839074587,4.17489652893168,22.7259383907459));
#12627=CARTESIAN_POINT('Ctrl Pts',(-2.70113892579397,4.16715584610488,22.7011399902602));
#12628=CARTESIAN_POINT('Ctrl Pts',(-2.675415676397,4.15846008560732,22.6754162485616));
#12629=CARTESIAN_POINT('Ctrl Pts',(-2.66426294033361,4.15468989622716,22.6642632990527));
#12630=CARTESIAN_POINT('Ctrl Pts',(-2.65293655145142,4.15073955259153,22.6529365514514));
#12631=CARTESIAN_POINT('Ctrl Pts',(-2.64142135623724,4.14658995368149,22.6414213562372));
#12632=CARTESIAN_POINT('',(-2.85857864376269,4.20972540916711,22.8585786437627));
#12633=CARTESIAN_POINT('Ctrl Pts',(-2.75,4.18187951621146,22.75));
#12634=CARTESIAN_POINT('Ctrl Pts',(-2.78604207307411,4.19233938758395,22.7860420730741));
#12635=CARTESIAN_POINT('Ctrl Pts',(-2.82223699994704,4.20161368298381,22.822236999947));
#12636=CARTESIAN_POINT('Ctrl Pts',(-2.85857864376269,4.20972540916711,22.8585786437627));
#12637=CARTESIAN_POINT('',(-2.85857864376269,7.275,22.8585786437627));
#12638=CARTESIAN_POINT('Ctrl Pts',(-3.90882250993909,3.66863444045392,21.6333060643901));
#12639=CARTESIAN_POINT('Ctrl Pts',(-1.59117749006091,3.66863444045392,21.6333060643901));
#12640=CARTESIAN_POINT('Ctrl Pts',(-3.90882250993909,3.86924203284188,22.0464620601053));
#12641=CARTESIAN_POINT('Ctrl Pts',(-1.59117749006091,3.86924203284188,22.0464620601053));
#12642=CARTESIAN_POINT('Ctrl Pts',(-3.90882250993909,4.06984962522984,22.4596180558205));
#12643=CARTESIAN_POINT('Ctrl Pts',(-1.59117749006091,4.06984962522984,22.4596180558205));
#12644=CARTESIAN_POINT('Ctrl Pts',(-3.90882250993909,4.25320571288467,22.8372441768646));
#12645=CARTESIAN_POINT('Ctrl Pts',(-1.59117749006091,4.25320571288467,22.8372441768646));
#12646=CARTESIAN_POINT('Ctrl Pts',(-3.90882250993909,4.25320571288467,23.2585265278816));
#12647=CARTESIAN_POINT('Ctrl Pts',(-1.59117749006091,4.25320571288467,23.2585265278816));
#12648=CARTESIAN_POINT('Ctrl Pts',(-3.90882250993909,4.25320571288467,23.6152196445594));
#12649=CARTESIAN_POINT('Ctrl Pts',(-1.59117749006091,4.25320571288467,23.6152196445594));
#12650=CARTESIAN_POINT('Ctrl Pts',(-3.90882250993909,4.25320571288467,23.9719127612371));
#12651=CARTESIAN_POINT('Ctrl Pts',(-1.59117749006091,4.25320571288467,23.9719127612371));
#12652=CARTESIAN_POINT('',(-2.75,4.22764086327576,22.95));
#12653=CARTESIAN_POINT('Ctrl Pts',(-2.61819805153246,4.14309288132937,22.6318019484625));
#12654=CARTESIAN_POINT('Ctrl Pts',(-2.66129757451431,4.1812519561426,22.735853401377));
#12655=CARTESIAN_POINT('Ctrl Pts',(-2.705238006854,4.20937166018217,22.8419349890681));
#12656=CARTESIAN_POINT('Ctrl Pts',(-2.74999999999719,4.22764086327461,22.9499999999932));
#12657=CARTESIAN_POINT('',(-2.75,4.25320571288467,23.2585265278816));
#12658=CARTESIAN_POINT('Ctrl Pts',(-2.75,4.22764086327576,22.95));
#12659=CARTESIAN_POINT('Ctrl Pts',(-2.75,4.25320571288467,23.101219828165));
#12660=CARTESIAN_POINT('Ctrl Pts',(-2.75,4.25320571288467,23.2585265278816));
#12661=CARTESIAN_POINT('',(-3.,4.25320571288467,23.2585265278816));
#12662=CARTESIAN_POINT('',(-3.,4.25320571288467,23.2585265278816));
#12663=CARTESIAN_POINT('',(-3.,4.25231459025407,23.2));
#12664=CARTESIAN_POINT('Ctrl Pts',(-3.,4.25231459025407,23.2));
#12665=CARTESIAN_POINT('Ctrl Pts',(-3.,4.25320571288467,23.2291571778681));
#12666=CARTESIAN_POINT('Ctrl Pts',(-3.,4.25320571288467,23.2585265278816));
#12667=CARTESIAN_POINT('Ctrl Pts',(-2.85857864376269,4.20972540916711,22.8585786437626));
#12668=CARTESIAN_POINT('Ctrl Pts',(-2.87504619169403,4.21859928476957,22.8983348213176));
#12669=CARTESIAN_POINT('Ctrl Pts',(-2.89164111829844,4.22611131569154,22.9383985181925));
#12670=CARTESIAN_POINT('Ctrl Pts',(-2.90836309848014,4.23226475621148,22.9787689495369));
#12671=CARTESIAN_POINT('Ctrl Pts',(-2.93876009161904,4.24345039853569,23.0521537826282));
#12672=CARTESIAN_POINT('Ctrl Pts',(-2.96931533762918,4.25005052457576,23.1259206719475));
#12673=CARTESIAN_POINT('Ctrl Pts',(-3.,4.25231459025406,23.2));
#12674=CARTESIAN_POINT('Origin',(-2.67928932188135,8.6365278666839,22.7792893218814));
#12675=CARTESIAN_POINT('',(-2.75,1.21971470205851,22.95));
#12676=CARTESIAN_POINT('Ctrl Pts',(-2.74999999998749,1.21971470206339,22.9499999999698));
#12677=CARTESIAN_POINT('Ctrl Pts',(-2.73139877750455,1.2269752233707,22.9050926763748));
#12678=CARTESIAN_POINT('Ctrl Pts',(-2.71230553313965,1.23602156967566,22.8590058283899));
#12679=CARTESIAN_POINT('Ctrl Pts',(-2.69279642154661,1.24726736451132,22.8119079585131));
#12680=CARTESIAN_POINT('Ctrl Pts',(-2.67356362688915,1.25835387974306,22.7654771584316));
#12681=CARTESIAN_POINT('Ctrl Pts',(-2.65392666183419,1.27157792698435,22.7180637445991));
#12682=CARTESIAN_POINT('Ctrl Pts',(-2.63395849080496,1.28738081230999,22.669852665828));
#12683=CARTESIAN_POINT('Ctrl Pts',(-2.62872730492721,1.29152079240241,22.6572225098638));
#12684=CARTESIAN_POINT('Ctrl Pts',(-2.62347338787422,1.2958380073702,22.6445377370048));
#12685=CARTESIAN_POINT('Ctrl Pts',(-2.61819805153393,1.30034092007739,22.631801948466));
#12686=CARTESIAN_POINT('',(-2.75,8.6365278666839,22.95));
#12687=CARTESIAN_POINT('Origin',(-2.92928932188134,-25.,26.5));
#12688=CARTESIAN_POINT('',(-2.85857864376269,-25.,29.6085786437627));
#12689=CARTESIAN_POINT('Origin',(-2.85857864376269,-25.,26.5));
#12690=CARTESIAN_POINT('',(-3.,-25.,29.95));
#12691=CARTESIAN_POINT('',(-2.92928932188134,-25.,29.7792893218813));
#12692=CARTESIAN_POINT('',(-3.,-23.9937694101251,23.2));
#12693=CARTESIAN_POINT('Origin',(-3.,-25.,26.5));
#12694=CARTESIAN_POINT('',(-2.96924080768304,-25.1,23.1257407407407));
#12695=CARTESIAN_POINT('Ctrl Pts',(-3.,-23.9937694101251,23.2));
#12696=CARTESIAN_POINT('Ctrl Pts',(-2.96584661721312,-24.5468847050626,
23.117546440075));
#12697=CARTESIAN_POINT('Ctrl Pts',(-2.96924080768304,-25.1,23.1257407407407));
#12698=CARTESIAN_POINT('',(-2.98964466094068,-28.425,26.5));
#12699=CARTESIAN_POINT('Ctrl Pts',(-2.96924080768304,-25.1,23.1257407407407));
#12700=CARTESIAN_POINT('Ctrl Pts',(-2.97167617572008,-25.496866151748,23.1316202392852));
#12701=CARTESIAN_POINT('Ctrl Pts',(-2.97423902617588,-25.9145067633212,
23.2113907046527));
#12702=CARTESIAN_POINT('Ctrl Pts',(-2.97919487113465,-26.7221083621966,
23.5339522011638));
#12703=CARTESIAN_POINT('Ctrl Pts',(-2.98155520782326,-27.1067474485937,
23.7906699067144));
#12704=CARTESIAN_POINT('Ctrl Pts',(-2.98530798368454,-27.7182976093007,
24.3894378387628));
#12705=CARTESIAN_POINT('Ctrl Pts',(-2.98694203866927,-27.9845822543924,
24.7719850468527));
#12706=CARTESIAN_POINT('Ctrl Pts',(-2.98911037827991,-28.337933609961,25.6124281223253));
#12707=CARTESIAN_POINT('Ctrl Pts',(-2.98964466094067,-28.425,26.0703241244361));
#12708=CARTESIAN_POINT('Ctrl Pts',(-2.98964466094067,-28.425,26.5));
#12709=CARTESIAN_POINT('',(-3.,-28.4,27.0852349955359));
#12710=CARTESIAN_POINT('Ctrl Pts',(-2.98964466094068,-28.425,26.5));
#12711=CARTESIAN_POINT('Ctrl Pts',(-2.98964466094068,-28.425,26.792617497768));
#12712=CARTESIAN_POINT('Ctrl Pts',(-3.,-28.4,27.0852349955359));
#12713=CARTESIAN_POINT('Origin',(-3.,-25.,26.5));
#12714=CARTESIAN_POINT('Origin',(-2.92928932188135,-25.1,26.5));
#12715=CARTESIAN_POINT('',(-3.,-25.1,23.2));
#12716=CARTESIAN_POINT('',(-2.85857864376269,-28.7414213562373,26.5));
#12717=CARTESIAN_POINT('Origin',(-2.85857864376269,-25.1,26.5));
#12718=CARTESIAN_POINT('',(-3.,-28.4,26.5));
#12719=CARTESIAN_POINT('Origin',(-2.92928932188134,7.275,23.0292893218813));
#12720=CARTESIAN_POINT('',(-3.,-4.03055921196938,23.2));
#12721=CARTESIAN_POINT('',(-3.,7.275,23.2));
#12722=CARTESIAN_POINT('',(-2.98084332489689,-4.03055921196938,23.1537516951561));
#12723=CARTESIAN_POINT('',(-3.02322456252495,-4.03055921196938,23.2560690538279));
#12724=CARTESIAN_POINT('',(-2.98084332489689,-2.52878561615944,23.1537516951561));
#12725=CARTESIAN_POINT('',(-2.98084332489689,1.62222039401531,23.1537516951561));
#12726=CARTESIAN_POINT('',(-2.9564690384473,-2.52878561615944,23.0949069622363));
#12727=CARTESIAN_POINT('Origin',(-2.225,-25.,26.5));
#12728=CARTESIAN_POINT('',(-1.45,-25.,28.2));
#12729=CARTESIAN_POINT('',(-2.225,-25.,28.975));
#12730=CARTESIAN_POINT('Origin',(-1.45,-25.,26.5));
#12731=CARTESIAN_POINT('Origin',(-2.92928932188134,25.,26.5));
#12732=CARTESIAN_POINT('',(-2.85857864376269,25.,29.6085786437627));
#12733=CARTESIAN_POINT('Origin',(-2.85857864376269,25.,26.5));
#12734=CARTESIAN_POINT('',(-3.00000000039677,25.,29.9500000009579));
#12735=CARTESIAN_POINT('',(-2.92928932188134,25.,29.7792893218813));
#12736=CARTESIAN_POINT('',(-3.,28.4,27.0852349955359));
#12737=CARTESIAN_POINT('Origin',(-3.,25.,26.5));
#12738=CARTESIAN_POINT('',(-2.98964466094067,28.425,26.5));
#12739=CARTESIAN_POINT('Ctrl Pts',(-3.,28.4,27.0852349955359));
#12740=CARTESIAN_POINT('Ctrl Pts',(-2.98964466094067,28.425,26.792617497768));
#12741=CARTESIAN_POINT('Ctrl Pts',(-2.98964466094067,28.425,26.5));
#12742=CARTESIAN_POINT('',(-2.96924080768304,25.1,23.1257407407407));
#12743=CARTESIAN_POINT('Ctrl Pts',(-2.98964466094067,28.425,26.5));
#12744=CARTESIAN_POINT('Ctrl Pts',(-2.98964466094067,28.425,26.0703241244361));
#12745=CARTESIAN_POINT('Ctrl Pts',(-2.98911037827991,28.337933609961,25.6124281223253));
#12746=CARTESIAN_POINT('Ctrl Pts',(-2.98694203866927,27.9845822543924,24.7719850468527));
#12747=CARTESIAN_POINT('Ctrl Pts',(-2.98530798368454,27.7182976093007,24.3894378387628));
#12748=CARTESIAN_POINT('Ctrl Pts',(-2.98155520782326,27.1067474485937,23.7906699067144));
#12749=CARTESIAN_POINT('Ctrl Pts',(-2.97919487113465,26.7221083621966,23.5339522011638));
#12750=CARTESIAN_POINT('Ctrl Pts',(-2.97423902617588,25.9145067633212,23.2113907046527));
#12751=CARTESIAN_POINT('Ctrl Pts',(-2.97167617572009,25.496866151748,23.1316202392852));
#12752=CARTESIAN_POINT('Ctrl Pts',(-2.96924080768304,25.1,23.1257407407407));
#12753=CARTESIAN_POINT('',(-3.,23.9937694101251,23.2));
#12754=CARTESIAN_POINT('Ctrl Pts',(-2.96924080768304,25.1,23.1257407407407));
#12755=CARTESIAN_POINT('Ctrl Pts',(-2.96584661719341,24.5468847018497,23.1175464400274));
#12756=CARTESIAN_POINT('Ctrl Pts',(-3.00000000039677,23.9937694036995,23.2000000009579));
#12757=CARTESIAN_POINT('Origin',(-3.,25.,26.5));
#12758=CARTESIAN_POINT('Origin',(-2.92928932188135,25.1,26.5));
#12759=CARTESIAN_POINT('',(-3.,28.4,26.5));
#12760=CARTESIAN_POINT('',(-3.,25.1,23.2));
#12761=CARTESIAN_POINT('Origin',(-2.92928932188134,28.5707106781187,52.5625));
#12762=CARTESIAN_POINT('',(-3.,28.4,65.9147650044641));
#12763=CARTESIAN_POINT('',(-3.,28.4,52.5625));
#12764=CARTESIAN_POINT('',(-2.98994700660664,28.4242700729927,66.6));
#12765=CARTESIAN_POINT('Ctrl Pts',(-2.98994700660664,28.4242700729927,66.6));
#12766=CARTESIAN_POINT('Ctrl Pts',(-2.98787522829607,28.4292717882883,66.2573825022345));
#12767=CARTESIAN_POINT('Ctrl Pts',(-3.,28.4,65.9147650044641));
#12768=CARTESIAN_POINT('',(-3.,28.4,66.6));
#12769=CARTESIAN_POINT('Origin',(-2.225,25.,26.5));
#12770=CARTESIAN_POINT('',(-1.45,25.,28.2));
#12771=CARTESIAN_POINT('',(-2.225,25.,28.975));
#12772=CARTESIAN_POINT('Origin',(-1.45,25.,26.5));
#12773=CARTESIAN_POINT('Origin',(-2.92928932188134,-25.,66.5));
#12774=CARTESIAN_POINT('',(-2.85857864376269,-25.,69.6085786437627));
#12775=CARTESIAN_POINT('Origin',(-2.85857864376269,-25.,66.5));
#12776=CARTESIAN_POINT('',(-2.9896446609407,-25.,69.9249999999999));
#12777=CARTESIAN_POINT('',(-2.92928932188134,-25.,69.7792893218814));
#12778=CARTESIAN_POINT('',(-3.,-24.4147650044641,69.9));
#12779=CARTESIAN_POINT('Ctrl Pts',(-2.9896446609407,-25.,69.9249999999999));
#12780=CARTESIAN_POINT('Ctrl Pts',(-2.98964466094078,-24.7073825022338,
69.9249999999997));
#12781=CARTESIAN_POINT('Ctrl Pts',(-3.,-24.4147650044641,69.9));
#12782=CARTESIAN_POINT('',(-3.,-28.4,65.9147650044641));
#12783=CARTESIAN_POINT('Origin',(-3.,-25.,66.5));
#12784=CARTESIAN_POINT('',(-2.98994700660664,-28.4242700729927,66.6));
#12785=CARTESIAN_POINT('Ctrl Pts',(-3.,-28.4,65.9147650044641));
#12786=CARTESIAN_POINT('Ctrl Pts',(-2.98787522829607,-28.4292717882883,
66.2573825022345));
#12787=CARTESIAN_POINT('Ctrl Pts',(-2.98994700660664,-28.4242700729927,
66.6));
#12788=CARTESIAN_POINT('',(-2.98994700660664,-25.1,69.9242700729927));
#12789=CARTESIAN_POINT('Ctrl Pts',(-2.98994700660664,-28.4242700729927,
66.6));
#12790=CARTESIAN_POINT('Ctrl Pts',(-2.99238240184869,-28.4183905087696,
67.0027501492822));
#12791=CARTESIAN_POINT('Ctrl Pts',(-2.99447851800497,-28.3364130892601,
67.4263094322197));
#12792=CARTESIAN_POINT('Ctrl Pts',(-2.99745891948881,-28.0052855480682,
68.2431214573392));
#12793=CARTESIAN_POINT('Ctrl Pts',(-2.99822330470336,-27.7420564500924,
68.6309143229168));
#12794=CARTESIAN_POINT('Ctrl Pts',(-2.99822330470336,-27.1309143229168,
69.2420564500924));
#12795=CARTESIAN_POINT('Ctrl Pts',(-2.99745891948882,-26.7431214573392,
69.5052855480682));
#12796=CARTESIAN_POINT('Ctrl Pts',(-2.99447851800497,-25.9263094322197,
69.8364130892601));
#12797=CARTESIAN_POINT('Ctrl Pts',(-2.99238240184869,-25.5027501492822,
69.9183905087696));
#12798=CARTESIAN_POINT('Ctrl Pts',(-2.98994700660664,-25.1,69.9242700729927));
#12799=CARTESIAN_POINT('Ctrl Pts',(-2.98994700660664,-25.1,69.9242700729927));
#12800=CARTESIAN_POINT('Ctrl Pts',(-2.98964466094069,-25.05,69.925));
#12801=CARTESIAN_POINT('Ctrl Pts',(-2.9896446609407,-25.,69.9249999999999));
#12802=CARTESIAN_POINT('Origin',(-2.92928932188134,-28.5707106781187,40.5375));
#12803=CARTESIAN_POINT('',(-2.85857864376269,-28.7414213562373,66.6));
#12804=CARTESIAN_POINT('',(-2.85857864376269,-28.7414213562373,40.5375));
#12805=CARTESIAN_POINT('',(-3.,-28.4,66.6));
#12806=CARTESIAN_POINT('',(-3.,-28.4,40.5375));
#12807=CARTESIAN_POINT('Origin',(-3.,0.,46.55));
#12808=CARTESIAN_POINT('',(-3.,24.4147650044641,69.9));
#12809=CARTESIAN_POINT('',(-3.,-7.275,69.9));
#12810=CARTESIAN_POINT('Origin',(-3.,25.,66.5));
#12811=CARTESIAN_POINT('',(-3.,7.275,23.2));
#12812=CARTESIAN_POINT('',(-3.,3.82537491619587,24.5060028672218));
#12813=CARTESIAN_POINT('Ctrl Pts',(-3.,4.25320571288467,23.2585265278816));
#12814=CARTESIAN_POINT('Ctrl Pts',(-3.,4.25320571288467,24.0552522778511));
#12815=CARTESIAN_POINT('Ctrl Pts',(-3.,3.82537491619587,24.5060028672218));
#12816=CARTESIAN_POINT('',(-3.,2.72087290883064,24.9567531585693));
#12817=CARTESIAN_POINT('Ctrl Pts',(-3.,3.82537491619587,24.5060028672218));
#12818=CARTESIAN_POINT('Ctrl Pts',(-3.,3.39754410088063,24.9567531585693));
#12819=CARTESIAN_POINT('Ctrl Pts',(-3.,2.72087290883064,24.9567531585693));
#12820=CARTESIAN_POINT('',(-3.,1.92196443676949,24.7450204730034));
#12821=CARTESIAN_POINT('Ctrl Pts',(-3.,2.72087290883064,24.9567531585693));
#12822=CARTESIAN_POINT('Ctrl Pts',(-3.,2.27776229381562,24.9567531585693));
#12823=CARTESIAN_POINT('Ctrl Pts',(-3.,1.92196443676949,24.7450204730034));
#12824=CARTESIAN_POINT('',(-3.,1.37953594326973,24.1545701563358));
#12825=CARTESIAN_POINT('Ctrl Pts',(-3.,1.92196443676949,24.7450204730034));
#12826=CARTESIAN_POINT('Ctrl Pts',(-3.,1.56616643071175,24.5332877874374));
#12827=CARTESIAN_POINT('Ctrl Pts',(-3.,1.37953594326973,24.1545701563358));
#12828=CARTESIAN_POINT('',(-3.,1.19290575385094,23.2956342935562));
#12829=CARTESIAN_POINT('Ctrl Pts',(-3.,1.37953594326973,24.1545701563358));
#12830=CARTESIAN_POINT('Ctrl Pts',(-3.,1.19290575385094,23.7758526742458));
#12831=CARTESIAN_POINT('Ctrl Pts',(-3.,1.19290575385094,23.2956342935562));
#12832=CARTESIAN_POINT('Ctrl Pts',(-3.,1.19290575385094,23.2956342935562));
#12833=CARTESIAN_POINT('Ctrl Pts',(-3.,1.19290575385094,23.1427574352851));
#12834=CARTESIAN_POINT('Ctrl Pts',(-3.,1.21228337796395,23.));
#12835=CARTESIAN_POINT('',(-3.,0.625375136733055,24.9));
#12836=CARTESIAN_POINT('',(-3.,0.625375136733055,34.1250000357628));
#12837=CARTESIAN_POINT('',(-3.,-1.5334241092205,24.9));
#12838=CARTESIAN_POINT('',(-3.,0.312687568366528,24.9));
#12839=CARTESIAN_POINT('',(-3.,-1.5334241092205,24.5223738789558));
#12840=CARTESIAN_POINT('',(-3.,-1.5334241092205,35.725));
#12841=CARTESIAN_POINT('',(-3.,0.201909989118576,24.5223738789558));
#12842=CARTESIAN_POINT('',(-3.,-0.766712054610252,24.5223738789558));
#12843=CARTESIAN_POINT('',(-3.,0.201909989118576,23.5313779652119));
#12844=CARTESIAN_POINT('',(-3.,0.201909989118576,35.5361869394779));
#12845=CARTESIAN_POINT('',(-3.,-1.29986360669136,23.5313779652119));
#12846=CARTESIAN_POINT('',(-3.,0.100954994559288,23.5313779652119));
#12847=CARTESIAN_POINT('',(-3.,-1.29986360669136,23.2));
#12848=CARTESIAN_POINT('',(-3.,-1.29986360669136,35.0406889826059));
#12849=CARTESIAN_POINT('',(-3.,-2.10532046854496,23.2));
#12850=CARTESIAN_POINT('',(-3.,7.275,23.2));
#12851=CARTESIAN_POINT('',(-3.,-2.10532046854496,24.9));
#12852=CARTESIAN_POINT('',(-3.,-2.10532046854496,34.1250000357628));
#12853=CARTESIAN_POINT('',(-3.,-4.26411971449852,24.9));
#12854=CARTESIAN_POINT('',(-3.,-1.05266023427248,24.9));
#12855=CARTESIAN_POINT('',(-3.,-4.26411971449852,24.5223738789558));
#12856=CARTESIAN_POINT('',(-3.,-4.26411971449852,35.725));
#12857=CARTESIAN_POINT('',(-3.,-2.52878561615944,24.5223738789558));
#12858=CARTESIAN_POINT('',(-3.,-2.13205985724926,24.5223738789558));
#12859=CARTESIAN_POINT('',(-3.,-2.52878561615944,23.5313779652119));
#12860=CARTESIAN_POINT('',(-3.,-2.52878561615944,35.5361869394779));
#12861=CARTESIAN_POINT('',(-3.,-4.03055921196938,23.5313779652119));
#12862=CARTESIAN_POINT('',(-3.,-1.26439280807972,23.5313779652119));
#12863=CARTESIAN_POINT('',(-3.,-4.03055921196938,35.0406889826059));
#12864=CARTESIAN_POINT('',(-3.,-4.03055921196938,65.1537516951561));
#12865=CARTESIAN_POINT('',(-3.,-2.52878561615944,65.1537516951561));
#12866=CARTESIAN_POINT('',(-3.,-2.01527960598469,65.1537516951561));
#12867=CARTESIAN_POINT('',(-3.,-2.52878561615944,63.7000000715256));
#12868=CARTESIAN_POINT('',(-3.,-2.52878561615944,55.851875847578));
#12869=CARTESIAN_POINT('',(-3.,-2.10532046854496,63.7000000715256));
#12870=CARTESIAN_POINT('',(-3.,-1.26439280807972,63.7000000715256));
#12871=CARTESIAN_POINT('',(-3.,-2.10532046854496,66.9));
#12872=CARTESIAN_POINT('',(-3.,-2.10532046854496,55.1250000357628));
#12873=CARTESIAN_POINT('',(-3.,-4.26411971449852,66.9));
#12874=CARTESIAN_POINT('',(-3.,-1.05266023427248,66.9));
#12875=CARTESIAN_POINT('',(-3.,-4.26411971449852,66.5223738789558));
#12876=CARTESIAN_POINT('',(-3.,-4.26411971449852,56.725));
#12877=CARTESIAN_POINT('',(-3.,-2.52878561615944,66.5223738789558));
#12878=CARTESIAN_POINT('',(-3.,-2.13205985724926,66.5223738789558));
#12879=CARTESIAN_POINT('',(-3.,-2.52878561615944,65.5313779652119));
#12880=CARTESIAN_POINT('',(-3.,-2.52878561615944,56.5361869394779));
#12881=CARTESIAN_POINT('',(-3.,-4.03055921196938,65.5313779652119));
#12882=CARTESIAN_POINT('',(-3.,-1.26439280807972,65.5313779652119));
#12883=CARTESIAN_POINT('',(-3.,-4.03055921196938,56.0406889826059));
#12884=CARTESIAN_POINT('',(-3.,-1.29986360669136,65.1537516951561));
#12885=CARTESIAN_POINT('',(-3.,0.201909989118576,65.1537516951561));
#12886=CARTESIAN_POINT('',(-3.,-0.64993180334568,65.1537516951561));
#12887=CARTESIAN_POINT('',(-3.,0.201909989118576,63.7000000715256));
#12888=CARTESIAN_POINT('',(-3.,0.201909989118576,55.851875847578));
#12889=CARTESIAN_POINT('',(-3.,0.625375136733055,63.7000000715256));
#12890=CARTESIAN_POINT('',(-3.,0.100954994559288,63.7000000715256));
#12891=CARTESIAN_POINT('',(-3.,0.625375136733055,66.9));
#12892=CARTESIAN_POINT('',(-3.,0.625375136733055,55.1250000357628));
#12893=CARTESIAN_POINT('',(-3.,-1.5334241092205,66.9));
#12894=CARTESIAN_POINT('',(-3.,0.312687568366528,66.9));
#12895=CARTESIAN_POINT('',(-3.,-1.5334241092205,66.5223738789558));
#12896=CARTESIAN_POINT('',(-3.,-1.5334241092205,56.725));
#12897=CARTESIAN_POINT('',(-3.,0.201909989118576,66.5223738789558));
#12898=CARTESIAN_POINT('',(-3.,-0.766712054610252,66.5223738789558));
#12899=CARTESIAN_POINT('',(-3.,0.201909989118576,65.5313779652119));
#12900=CARTESIAN_POINT('',(-3.,0.201909989118576,56.5361869394779));
#12901=CARTESIAN_POINT('',(-3.,-1.29986360669136,65.5313779652119));
#12902=CARTESIAN_POINT('',(-3.,0.100954994559288,65.5313779652119));
#12903=CARTESIAN_POINT('',(-3.,-1.29986360669136,56.0406889826059));
#12904=CARTESIAN_POINT('',(-3.,2.72305563092232,63.6454299330711));
#12905=CARTESIAN_POINT('',(-3.,3.53069551289082,63.8637107849121));
#12906=CARTESIAN_POINT('Ctrl Pts',(-3.,2.72305563092232,63.6454299330711));
#12907=CARTESIAN_POINT('Ctrl Pts',(-3.,3.17489743232727,63.6454299330711));
#12908=CARTESIAN_POINT('Ctrl Pts',(-3.,3.53069551289082,63.8637107849121));
#12909=CARTESIAN_POINT('',(-3.,4.06984962522984,64.4596180558205));
#12910=CARTESIAN_POINT('Ctrl Pts',(-3.,3.53069551289082,63.8637107849121));
#12911=CARTESIAN_POINT('Ctrl Pts',(-3.,3.88649359345436,64.0819919347763));
#12912=CARTESIAN_POINT('Ctrl Pts',(-3.,4.06984962522984,64.4596180558205));
#12913=CARTESIAN_POINT('',(-3.,4.25320571288467,65.2585265278816));
#12914=CARTESIAN_POINT('Ctrl Pts',(-3.,4.06984962522984,64.4596180558205));
#12915=CARTESIAN_POINT('Ctrl Pts',(-3.,4.25320571288467,64.8372441768646));
#12916=CARTESIAN_POINT('Ctrl Pts',(-3.,4.25320571288467,65.2585265278816));
#12917=CARTESIAN_POINT('',(-3.,3.82537491619587,66.5060028672218));
#12918=CARTESIAN_POINT('Ctrl Pts',(-3.,4.25320571288467,65.2585265278816));
#12919=CARTESIAN_POINT('Ctrl Pts',(-3.,4.25320571288467,66.0552522778511));
#12920=CARTESIAN_POINT('Ctrl Pts',(-3.,3.82537491619587,66.5060028672218));
#12921=CARTESIAN_POINT('',(-3.,2.72087290883064,66.9567531585693));
#12922=CARTESIAN_POINT('Ctrl Pts',(-3.,3.82537491619587,66.5060028672218));
#12923=CARTESIAN_POINT('Ctrl Pts',(-3.,3.39754410088063,66.9567531585693));
#12924=CARTESIAN_POINT('Ctrl Pts',(-3.,2.72087290883064,66.9567531585693));
#12925=CARTESIAN_POINT('',(-3.,1.92196443676949,66.7450204730034));
#12926=CARTESIAN_POINT('Ctrl Pts',(-3.,2.72087290883064,66.9567531585693));
#12927=CARTESIAN_POINT('Ctrl Pts',(-3.,2.27776229381562,66.9567531585693));
#12928=CARTESIAN_POINT('Ctrl Pts',(-3.,1.92196443676949,66.7450204730034));
#12929=CARTESIAN_POINT('',(-3.,1.37953594326973,66.1545701563358));
#12930=CARTESIAN_POINT('Ctrl Pts',(-3.,1.92196443676949,66.7450204730034));
#12931=CARTESIAN_POINT('Ctrl Pts',(-3.,1.56616643071175,66.5332877874374));
#12932=CARTESIAN_POINT('Ctrl Pts',(-3.,1.37953594326973,66.1545701563358));
#12933=CARTESIAN_POINT('',(-3.,1.19290575385094,65.2956342935562));
#12934=CARTESIAN_POINT('Ctrl Pts',(-3.,1.37953594326973,66.1545701563358));
#12935=CARTESIAN_POINT('Ctrl Pts',(-3.,1.19290575385094,65.7758526742458));
#12936=CARTESIAN_POINT('Ctrl Pts',(-3.,1.19290575385094,65.2956342935562));
#12937=CARTESIAN_POINT('',(-3.,1.38935878872872,64.4246930122376));
#12938=CARTESIAN_POINT('Ctrl Pts',(-3.,1.19290575385094,65.2956342935562));
#12939=CARTESIAN_POINT('Ctrl Pts',(-3.,1.19290575385094,64.80886759758));
#12940=CARTESIAN_POINT('Ctrl Pts',(-3.,1.38935878872872,64.4246930122376));
#12941=CARTESIAN_POINT('',(-3.,1.94597527384758,63.8429740309715));
#12942=CARTESIAN_POINT('Ctrl Pts',(-3.,1.38935878872872,64.4246930122376));
#12943=CARTESIAN_POINT('Ctrl Pts',(-3.,1.58581152558327,64.0405184268951));
#12944=CARTESIAN_POINT('Ctrl Pts',(-3.,1.94597527384758,63.8429740309715));
#12945=CARTESIAN_POINT('Ctrl Pts',(-3.,1.94597527384758,63.8429740309715));
#12946=CARTESIAN_POINT('Ctrl Pts',(-3.,2.30613887310028,63.6454299330711));
#12947=CARTESIAN_POINT('Ctrl Pts',(-3.,2.72305563092232,63.6454299330711));
#12948=CARTESIAN_POINT('',(-3.,-22.6896318495274,41.4999999403954));
#12949=CARTESIAN_POINT('',(-3.,-20.5886767506599,44.6432467103004));
#12950=CARTESIAN_POINT('',(-3.,-18.0197882014912,48.4865704628042));
#12951=CARTESIAN_POINT('',(-3.,-20.5886767506599,41.4999999403954));
#12952=CARTESIAN_POINT('',(-3.,-20.5886767506599,45.5966233551502));
#12953=CARTESIAN_POINT('',(-3.,-20.0811733752489,41.4999999403954));
#12954=CARTESIAN_POINT('',(-3.,-10.29433837533,41.4999999403953));
#12955=CARTESIAN_POINT('',(-3.,-20.0811733752489,45.5));
#12956=CARTESIAN_POINT('',(-3.,-20.0811733752489,44.0249999701977));
#12957=CARTESIAN_POINT('',(-3.,-20.6241474747658,45.5));
#12958=CARTESIAN_POINT('',(-3.,-10.0405866876245,45.5));
#12959=CARTESIAN_POINT('',(-3.,-22.7251025736332,42.3594816327095));
#12960=CARTESIAN_POINT('',(-3.,-17.1933097703598,50.6284336498615));
#12961=CARTESIAN_POINT('',(-3.,-22.7251025736332,45.5));
#12962=CARTESIAN_POINT('',(-3.,-22.7251025736332,44.4547408163547));
#12963=CARTESIAN_POINT('',(-3.,-23.2326057255268,45.5));
#12964=CARTESIAN_POINT('',(-3.,-11.3625512868166,45.5));
#12965=CARTESIAN_POINT('',(-3.,-23.2326057255268,41.4999999403954));
#12966=CARTESIAN_POINT('',(-3.,-23.2326057255268,46.025));
#12967=CARTESIAN_POINT('',(-3.,-11.6163028627634,41.4999999403953));
#12968=CARTESIAN_POINT('',(-3.,-17.4918144643307,41.4317871928215));
#12969=CARTESIAN_POINT('',(-3.,-16.4822646677494,41.7046384811401));
#12970=CARTESIAN_POINT('Ctrl Pts',(-3.,-17.4918144643307,41.4317871928215));
#12971=CARTESIAN_POINT('Ctrl Pts',(-3.,-16.9270123243332,41.4317871928215));
#12972=CARTESIAN_POINT('Ctrl Pts',(-3.,-16.4822646677494,41.7046384811401));
#12973=CARTESIAN_POINT('',(-3.,-15.8083220273256,42.4495224952698));
#12974=CARTESIAN_POINT('Ctrl Pts',(-3.,-16.4822646677494,41.7046384811401));
#12975=CARTESIAN_POINT('Ctrl Pts',(-3.,-16.0375170856714,41.9774897694588));
#12976=CARTESIAN_POINT('Ctrl Pts',(-3.,-15.8083220273256,42.4495224952698));
#12977=CARTESIAN_POINT('',(-3.,-15.5791269317269,43.4481580853462));
#12978=CARTESIAN_POINT('Ctrl Pts',(-3.,-15.8083220273256,42.4495224952698));
#12979=CARTESIAN_POINT('Ctrl Pts',(-3.,-15.5791269317269,42.9215552210808));
#12980=CARTESIAN_POINT('Ctrl Pts',(-3.,-15.5791269317269,43.4481580853462));
#12981=CARTESIAN_POINT('',(-3.,-16.1139154136181,45.0075035095215));
#12982=CARTESIAN_POINT('Ctrl Pts',(-3.,-15.5791269317269,43.4481580853462));
#12983=CARTESIAN_POINT('Ctrl Pts',(-3.,-15.5791269317269,44.4440655708313));
#12984=CARTESIAN_POINT('Ctrl Pts',(-3.,-16.1139154136181,45.0075035095215));
#12985=CARTESIAN_POINT('',(-3.,-17.4945430159569,45.5709411501884));
#12986=CARTESIAN_POINT('Ctrl Pts',(-3.,-16.1139154136181,45.0075035095215));
#12987=CARTESIAN_POINT('Ctrl Pts',(-3.,-16.6487039327621,45.5709411501884));
#12988=CARTESIAN_POINT('Ctrl Pts',(-3.,-17.4945430159569,45.5709411501884));
#12989=CARTESIAN_POINT('',(-3.,-18.4931787550449,45.30627566576));
#12990=CARTESIAN_POINT('Ctrl Pts',(-3.,-17.4945430159569,45.5709411501884));
#12991=CARTESIAN_POINT('Ctrl Pts',(-3.,-18.0484312474728,45.5709411501884));
#12992=CARTESIAN_POINT('Ctrl Pts',(-3.,-18.4931787550449,45.30627566576));
#12993=CARTESIAN_POINT('',(-3.,-19.1712143719196,44.5682128071785));
#12994=CARTESIAN_POINT('Ctrl Pts',(-3.,-18.4931787550449,45.30627566576));
#12995=CARTESIAN_POINT('Ctrl Pts',(-3.,-18.9379265606403,45.0416098833084));
#12996=CARTESIAN_POINT('Ctrl Pts',(-3.,-19.1712143719196,44.5682128071785));
#12997=CARTESIAN_POINT('',(-3.,-19.4045021831989,43.4945430159569));
#12998=CARTESIAN_POINT('Ctrl Pts',(-3.,-19.1712143719196,44.5682128071785));
#12999=CARTESIAN_POINT('Ctrl Pts',(-3.,-19.4045021831989,44.0948157310486));
#13000=CARTESIAN_POINT('Ctrl Pts',(-3.,-19.4045021831989,43.4945430159569));
#13001=CARTESIAN_POINT('',(-3.,-19.1589361131191,42.4058662652969));
#13002=CARTESIAN_POINT('Ctrl Pts',(-3.,-19.4045021831989,43.4945430159569));
#13003=CARTESIAN_POINT('Ctrl Pts',(-3.,-19.4045021831989,42.8860844969749));
#13004=CARTESIAN_POINT('Ctrl Pts',(-3.,-19.1589361131191,42.4058662652969));
#13005=CARTESIAN_POINT('',(-3.,-18.4631651341915,41.6787176132202));
#13006=CARTESIAN_POINT('Ctrl Pts',(-3.,-19.1589361131191,42.4058662652969));
#13007=CARTESIAN_POINT('Ctrl Pts',(-3.,-18.9133697450161,41.9256480336189));
#13008=CARTESIAN_POINT('Ctrl Pts',(-3.,-18.4631651341915,41.6787176132202));
#13009=CARTESIAN_POINT('Ctrl Pts',(-3.,-18.4631651341915,41.6787176132202));
#13010=CARTESIAN_POINT('Ctrl Pts',(-3.,-18.0129605233669,41.4317871928215));
#13011=CARTESIAN_POINT('Ctrl Pts',(-3.,-17.4918144643307,41.4317871928215));
#13012=CARTESIAN_POINT('',(-3.,-7.9602041944578E-16,54.));
#13013=CARTESIAN_POINT('Origin',(-3.,0.,47.5));
#13014=CARTESIAN_POINT('',(-3.,21.5081855356693,41.4317871928215));
#13015=CARTESIAN_POINT('',(-3.,22.5177353322506,41.7046384811401));
#13016=CARTESIAN_POINT('Ctrl Pts',(-3.,21.5081855356693,41.4317871928215));
#13017=CARTESIAN_POINT('Ctrl Pts',(-3.,22.0729876756668,41.4317871928215));
#13018=CARTESIAN_POINT('Ctrl Pts',(-3.,22.5177353322506,41.7046384811401));
#13019=CARTESIAN_POINT('',(-3.,23.1916779726744,42.4495224952698));
#13020=CARTESIAN_POINT('Ctrl Pts',(-3.,22.5177353322506,41.7046384811401));
#13021=CARTESIAN_POINT('Ctrl Pts',(-3.,22.9624829143286,41.9774897694588));
#13022=CARTESIAN_POINT('Ctrl Pts',(-3.,23.1916779726744,42.4495224952698));
#13023=CARTESIAN_POINT('',(-3.,23.4208730682731,43.4481580853462));
#13024=CARTESIAN_POINT('Ctrl Pts',(-3.,23.1916779726744,42.4495224952698));
#13025=CARTESIAN_POINT('Ctrl Pts',(-3.,23.4208730682731,42.9215552210808));
#13026=CARTESIAN_POINT('Ctrl Pts',(-3.,23.4208730682731,43.4481580853462));
#13027=CARTESIAN_POINT('',(-3.,22.8860845863819,45.0075035095215));
#13028=CARTESIAN_POINT('Ctrl Pts',(-3.,23.4208730682731,43.4481580853462));
#13029=CARTESIAN_POINT('Ctrl Pts',(-3.,23.4208730682731,44.4440655708313));
#13030=CARTESIAN_POINT('Ctrl Pts',(-3.,22.8860845863819,45.0075035095215));
#13031=CARTESIAN_POINT('',(-3.,21.5054569840431,45.5709411501884));
#13032=CARTESIAN_POINT('Ctrl Pts',(-3.,22.8860845863819,45.0075035095215));
#13033=CARTESIAN_POINT('Ctrl Pts',(-3.,22.3512960672379,45.5709411501884));
#13034=CARTESIAN_POINT('Ctrl Pts',(-3.,21.5054569840431,45.5709411501884));
#13035=CARTESIAN_POINT('',(-3.,20.5068212449551,45.30627566576));
#13036=CARTESIAN_POINT('Ctrl Pts',(-3.,21.5054569840431,45.5709411501884));
#13037=CARTESIAN_POINT('Ctrl Pts',(-3.,20.9515687525272,45.5709411501884));
#13038=CARTESIAN_POINT('Ctrl Pts',(-3.,20.5068212449551,45.30627566576));
#13039=CARTESIAN_POINT('',(-3.,19.8287856280804,44.5682128071785));
#13040=CARTESIAN_POINT('Ctrl Pts',(-3.,20.5068212449551,45.30627566576));
#13041=CARTESIAN_POINT('Ctrl Pts',(-3.,20.0620734393597,45.0416098833084));
#13042=CARTESIAN_POINT('Ctrl Pts',(-3.,19.8287856280804,44.5682128071785));
#13043=CARTESIAN_POINT('',(-3.,19.5954978168011,43.4945430159569));
#13044=CARTESIAN_POINT('Ctrl Pts',(-3.,19.8287856280804,44.5682128071785));
#13045=CARTESIAN_POINT('Ctrl Pts',(-3.,19.5954978168011,44.0948157310486));
#13046=CARTESIAN_POINT('Ctrl Pts',(-3.,19.5954978168011,43.4945430159569));
#13047=CARTESIAN_POINT('',(-3.,19.8410638868809,42.4058662652969));
#13048=CARTESIAN_POINT('Ctrl Pts',(-3.,19.5954978168011,43.4945430159569));
#13049=CARTESIAN_POINT('Ctrl Pts',(-3.,19.5954978168011,42.8860844969749));
#13050=CARTESIAN_POINT('Ctrl Pts',(-3.,19.8410638868809,42.4058662652969));
#13051=CARTESIAN_POINT('',(-3.,20.5368348658085,41.6787176132202));
#13052=CARTESIAN_POINT('Ctrl Pts',(-3.,19.8410638868809,42.4058662652969));
#13053=CARTESIAN_POINT('Ctrl Pts',(-3.,20.0866302549839,41.9256480336189));
#13054=CARTESIAN_POINT('Ctrl Pts',(-3.,20.5368348658085,41.6787176132202));
#13055=CARTESIAN_POINT('Ctrl Pts',(-3.,20.5368348658085,41.6787176132202));
#13056=CARTESIAN_POINT('Ctrl Pts',(-3.,20.9870394766331,41.4317871928215));
#13057=CARTESIAN_POINT('Ctrl Pts',(-3.,21.5081855356693,41.4317871928215));
#13058=CARTESIAN_POINT('',(-3.,16.3103681504726,41.4999999403954));
#13059=CARTESIAN_POINT('',(-3.,18.4113232493401,44.6432467103004));
#13060=CARTESIAN_POINT('',(-3.,14.9585828206595,39.4775888599155));
#13061=CARTESIAN_POINT('',(-3.,18.4113232493401,41.4999999403954));
#13062=CARTESIAN_POINT('',(-3.,18.4113232493401,45.5966233551502));
#13063=CARTESIAN_POINT('',(-3.,18.9188266247511,41.4999999403954));
#13064=CARTESIAN_POINT('',(-3.,9.20566162467003,41.4999999403953));
#13065=CARTESIAN_POINT('',(-3.,18.9188266247511,45.5));
#13066=CARTESIAN_POINT('',(-3.,18.9188266247511,44.0249999701977));
#13067=CARTESIAN_POINT('',(-3.,18.3758525252342,45.5));
#13068=CARTESIAN_POINT('',(-3.,9.45941331237555,45.5));
#13069=CARTESIAN_POINT('',(-3.,16.2748974263668,42.3594816327095));
#13070=CARTESIAN_POINT('',(-3.,15.777830067132,41.6164628160299));
#13071=CARTESIAN_POINT('',(-3.,16.2748974263668,45.5));
#13072=CARTESIAN_POINT('',(-3.,16.2748974263668,44.4547408163547));
#13073=CARTESIAN_POINT('',(-3.,15.7673942744732,45.5));
#13074=CARTESIAN_POINT('',(-3.,8.1374487131834,45.5));
#13075=CARTESIAN_POINT('',(-3.,15.7673942744732,41.4999999403954));
#13076=CARTESIAN_POINT('',(-3.,15.7673942744732,46.025));
#13077=CARTESIAN_POINT('',(-3.,7.8836971372366,41.4999999403953));
#13078=CARTESIAN_POINT('Origin',(-2.225,-25.,66.5));
#13079=CARTESIAN_POINT('',(-1.45,-25.,68.2));
#13080=CARTESIAN_POINT('',(-2.225,-25.,68.975));
#13081=CARTESIAN_POINT('Origin',(-1.45,-25.,66.5));
#13082=CARTESIAN_POINT('Origin',(-2.92928932188134,25.,66.5));
#13083=CARTESIAN_POINT('',(-2.85857864376269,25.,69.6085786437627));
#13084=CARTESIAN_POINT('Origin',(-2.85857864376269,25.,66.5));
#13085=CARTESIAN_POINT('',(-2.9896446609407,25.,69.9249999999999));
#13086=CARTESIAN_POINT('',(-2.92928932188134,25.,69.7792893218814));
#13087=CARTESIAN_POINT('',(-2.98994700660664,25.1,69.9242700729927));
#13088=CARTESIAN_POINT('Ctrl Pts',(-2.9896446609407,25.,69.9249999999999));
#13089=CARTESIAN_POINT('Ctrl Pts',(-2.98964466094069,25.0500000000001,69.925));
#13090=CARTESIAN_POINT('Ctrl Pts',(-2.98994700660664,25.1,69.9242700729927));
#13091=CARTESIAN_POINT('Ctrl Pts',(-2.98994700660664,25.1,69.9242700729927));
#13092=CARTESIAN_POINT('Ctrl Pts',(-2.99238240184869,25.5027501492823,69.9183905087696));
#13093=CARTESIAN_POINT('Ctrl Pts',(-2.99447851800497,25.9263094322197,69.8364130892601));
#13094=CARTESIAN_POINT('Ctrl Pts',(-2.99745891948881,26.7431214573392,69.5052855480682));
#13095=CARTESIAN_POINT('Ctrl Pts',(-2.99822330470336,27.1309143229168,69.2420564500924));
#13096=CARTESIAN_POINT('Ctrl Pts',(-2.99822330470336,27.7420564500924,68.6309143229168));
#13097=CARTESIAN_POINT('Ctrl Pts',(-2.99745891948881,28.0052855480682,68.2431214573392));
#13098=CARTESIAN_POINT('Ctrl Pts',(-2.99447851800497,28.3364130892601,67.4263094322197));
#13099=CARTESIAN_POINT('Ctrl Pts',(-2.99238240184869,28.4183905087696,67.0027501492822));
#13100=CARTESIAN_POINT('Ctrl Pts',(-2.98994700660664,28.4242700729927,66.6));
#13101=CARTESIAN_POINT('Ctrl Pts',(-3.,24.4147650044641,69.9));
#13102=CARTESIAN_POINT('Ctrl Pts',(-2.98964466094078,24.7073825022338,69.9249999999997));
#13103=CARTESIAN_POINT('Ctrl Pts',(-2.9896446609407,25.,69.9249999999999));
#13104=CARTESIAN_POINT('Origin',(-2.225,25.,66.5));
#13105=CARTESIAN_POINT('',(-1.45,25.,68.2));
#13106=CARTESIAN_POINT('',(-2.225,25.,68.975));
#13107=CARTESIAN_POINT('Origin',(-1.45,25.,66.5));
#13108=CARTESIAN_POINT('Origin',(-2.92928932188134,7.275,23.0292893218813));
#13109=CARTESIAN_POINT('',(-2.69947963063977,-2.10532046854496,22.4744796485212));
#13110=CARTESIAN_POINT('',(-2.98084332489689,-1.29986360669136,23.1537516951561));
#13111=CARTESIAN_POINT('',(-3.02322456252495,-1.29986360669136,23.2560690538279));
#13112=CARTESIAN_POINT('',(-2.98084332489689,0.201909989118576,23.1537516951561));
#13113=CARTESIAN_POINT('',(-2.98084332489689,2.98756819665432,23.1537516951561));
#13114=CARTESIAN_POINT('',(-2.9564690384473,0.201909989118577,23.0949069622363));
#13115=CARTESIAN_POINT('Origin',(-3.,0.201909989118576,23.1537516951561));
#13116=CARTESIAN_POINT('',(-2.75,0.201909989118576,23.1537516951561));
#13117=CARTESIAN_POINT('',(-3.,0.201909989118576,23.1537516951561));
#13118=CARTESIAN_POINT('',(-2.75,0.201909989118576,23.1537516951561));
#13119=CARTESIAN_POINT('Origin',(-3.,-1.29986360669136,23.1537516951561));
#13120=CARTESIAN_POINT('',(-2.75,-1.29986360669136,23.1537516951561));
#13121=CARTESIAN_POINT('',(-3.,-1.29986360669136,23.1537516951561));
#13122=CARTESIAN_POINT('',(-2.75,-1.29986360669136,23.1537516951561));
#13123=CARTESIAN_POINT('Origin',(-2.92928932188134,7.275,23.0292893218813));
#13124=CARTESIAN_POINT('Origin',(-2.92928932188134,25.1,66.6));
#13125=CARTESIAN_POINT('',(-3.,25.1,69.9));
#13126=CARTESIAN_POINT('Origin',(-2.92928932188135,-7.275,70.0707106781187));
#13127=CARTESIAN_POINT('',(-2.85857864376268,-25.1,70.2414213562373));
#13128=CARTESIAN_POINT('',(-3.,-25.1,69.9));
#13129=CARTESIAN_POINT('',(-2.85857864376269,-7.275,70.2414213562373));
#13130=CARTESIAN_POINT('Origin',(-2.92928932188135,-25.1,66.6));
#13131=CARTESIAN_POINT('Origin',(-2.85857864376269,-25.1,66.6));
#13132=CARTESIAN_POINT('Origin',(-2.75,-14.55,70.35));
#13133=CARTESIAN_POINT('',(-2.5,-25.1,70.6));
#13134=CARTESIAN_POINT('Origin',(-2.75,-25.1,66.6));
#13135=CARTESIAN_POINT('',(-3.,-28.6,66.6));
#13136=CARTESIAN_POINT('Origin',(-2.75,-28.85,34.525));
#13137=CARTESIAN_POINT('',(-3.,-28.6,26.5));
#13138=CARTESIAN_POINT('Origin',(-2.75,-25.1,26.5));
#13139=CARTESIAN_POINT('Origin',(-3.,-2.52878561615944,23.1537516951561));
#13140=CARTESIAN_POINT('',(-2.75,-2.52878561615944,23.1537516951561));
#13141=CARTESIAN_POINT('',(-3.,-2.52878561615944,23.1537516951561));
#13142=CARTESIAN_POINT('',(-2.75,-2.52878561615944,23.1537516951561));
#13143=CARTESIAN_POINT('Origin',(-3.,-4.03055921196938,23.1537516951561));
#13144=CARTESIAN_POINT('',(-2.75,-4.03055921196938,23.1537516951561));
#13145=CARTESIAN_POINT('',(-3.,-4.03055921196938,23.1537516951561));
#13146=CARTESIAN_POINT('',(-2.75,-4.03055921196938,23.1537516951561));
#13147=CARTESIAN_POINT('Origin',(-2.75,2.7230557333678,23.3010915458202));
#13148=CARTESIAN_POINT('',(-2.75,1.19290575385094,23.2956342935562));
#13149=CARTESIAN_POINT('Ctrl Pts',(-2.75,1.19290575385094,23.2956342935562));
#13150=CARTESIAN_POINT('Ctrl Pts',(-2.75,1.19290575385094,23.1158170345574));
#13151=CARTESIAN_POINT('Ctrl Pts',(-2.75,1.21971470205851,22.95));
#13152=CARTESIAN_POINT('',(-2.75,1.37953594326973,24.1545701563358));
#13153=CARTESIAN_POINT('Ctrl Pts',(-2.75,1.37953594326973,24.1545701563358));
#13154=CARTESIAN_POINT('Ctrl Pts',(-2.75,1.19290575385094,23.7758526742458));
#13155=CARTESIAN_POINT('Ctrl Pts',(-2.75,1.19290575385094,23.2956342935562));
#13156=CARTESIAN_POINT('',(-2.75,1.92196443676949,24.7450204730034));
#13157=CARTESIAN_POINT('Ctrl Pts',(-2.75,1.92196443676949,24.7450204730034));
#13158=CARTESIAN_POINT('Ctrl Pts',(-2.75,1.56616643071175,24.5332877874374));
#13159=CARTESIAN_POINT('Ctrl Pts',(-2.75,1.37953594326973,24.1545701563358));
#13160=CARTESIAN_POINT('',(-2.75,2.72087290883064,24.9567531585693));
#13161=CARTESIAN_POINT('Ctrl Pts',(-2.75,2.72087290883064,24.9567531585693));
#13162=CARTESIAN_POINT('Ctrl Pts',(-2.75,2.27776229381562,24.9567531585693));
#13163=CARTESIAN_POINT('Ctrl Pts',(-2.75,1.92196443676949,24.7450204730034));
#13164=CARTESIAN_POINT('',(-2.75,3.82537491619587,24.5060028672218));
#13165=CARTESIAN_POINT('Ctrl Pts',(-2.75,3.82537491619587,24.5060028672218));
#13166=CARTESIAN_POINT('Ctrl Pts',(-2.75,3.39754410088063,24.9567531585693));
#13167=CARTESIAN_POINT('Ctrl Pts',(-2.75,2.72087290883064,24.9567531585693));
#13168=CARTESIAN_POINT('Ctrl Pts',(-2.75,4.25320571288467,23.2585265278816));
#13169=CARTESIAN_POINT('Ctrl Pts',(-2.75,4.25320571288467,24.0552522778511));
#13170=CARTESIAN_POINT('Ctrl Pts',(-2.75,3.82537491619587,24.5060028672218));
#13171=CARTESIAN_POINT('Origin',(-3.,-4.03055921196938,23.5313779652119));
#13172=CARTESIAN_POINT('',(-2.75,-4.03055921196938,23.5313779652119));
#13173=CARTESIAN_POINT('',(-3.,-4.03055921196938,23.5313779652119));
#13174=CARTESIAN_POINT('',(-2.75,-4.03055921196938,23.5313779652119));
#13175=CARTESIAN_POINT('Origin',(-3.,-2.52878561615944,23.5313779652119));
#13176=CARTESIAN_POINT('',(-2.75,-2.52878561615944,23.5313779652119));
#13177=CARTESIAN_POINT('',(-3.,-2.52878561615944,23.5313779652119));
#13178=CARTESIAN_POINT('',(-2.75,-2.52878561615944,23.5313779652119));
#13179=CARTESIAN_POINT('Origin',(-3.,-2.52878561615944,24.5223738789558));
#13180=CARTESIAN_POINT('',(-2.75,-2.52878561615944,24.5223738789558));
#13181=CARTESIAN_POINT('',(-3.,-2.52878561615944,24.5223738789558));
#13182=CARTESIAN_POINT('',(-2.75,-2.52878561615944,24.5223738789558));
#13183=CARTESIAN_POINT('Origin',(-3.,-4.26411971449852,24.5223738789558));
#13184=CARTESIAN_POINT('',(-2.75,-4.26411971449852,24.5223738789558));
#13185=CARTESIAN_POINT('',(-3.,-4.26411971449852,24.5223738789558));
#13186=CARTESIAN_POINT('',(-2.75,-4.26411971449852,24.5223738789558));
#13187=CARTESIAN_POINT('Origin',(-3.,-4.26411971449852,24.9));
#13188=CARTESIAN_POINT('',(-2.75,-4.26411971449852,24.9));
#13189=CARTESIAN_POINT('',(-3.,-4.26411971449852,24.9));
#13190=CARTESIAN_POINT('',(-2.75,-4.26411971449852,24.9));
#13191=CARTESIAN_POINT('Origin',(-3.,-2.10532046854496,24.9));
#13192=CARTESIAN_POINT('',(-2.75,-2.10532046854496,24.9));
#13193=CARTESIAN_POINT('',(-3.,-2.10532046854496,24.9));
#13194=CARTESIAN_POINT('',(-2.75,-2.10532046854496,24.9));
#13195=CARTESIAN_POINT('Origin',(-3.,-2.10532046854496,21.7000000715256));
#13196=CARTESIAN_POINT('',(-2.75,-2.10532046854496,21.7000000715256));
#13197=CARTESIAN_POINT('Origin',(-2.75,-3.18472009152174,23.3000000357628));
#13198=CARTESIAN_POINT('Origin',(-3.,-1.29986360669136,23.5313779652119));
#13199=CARTESIAN_POINT('',(-2.75,-1.29986360669136,23.5313779652119));
#13200=CARTESIAN_POINT('',(-3.,-1.29986360669136,23.5313779652119));
#13201=CARTESIAN_POINT('',(-2.75,-1.29986360669136,23.5313779652119));
#13202=CARTESIAN_POINT('Origin',(-3.,0.201909989118576,23.5313779652119));
#13203=CARTESIAN_POINT('',(-2.75,0.201909989118576,23.5313779652119));
#13204=CARTESIAN_POINT('',(-3.,0.201909989118576,23.5313779652119));
#13205=CARTESIAN_POINT('',(-2.75,0.201909989118576,23.5313779652119));
#13206=CARTESIAN_POINT('Origin',(-3.,0.201909989118576,24.5223738789558));
#13207=CARTESIAN_POINT('',(-2.75,0.201909989118576,24.5223738789558));
#13208=CARTESIAN_POINT('',(-3.,0.201909989118576,24.5223738789558));
#13209=CARTESIAN_POINT('',(-2.75,0.201909989118576,24.5223738789558));
#13210=CARTESIAN_POINT('Origin',(-3.,-1.5334241092205,24.5223738789558));
#13211=CARTESIAN_POINT('',(-2.75,-1.5334241092205,24.5223738789558));
#13212=CARTESIAN_POINT('',(-3.,-1.5334241092205,24.5223738789558));
#13213=CARTESIAN_POINT('',(-2.75,-1.5334241092205,24.5223738789558));
#13214=CARTESIAN_POINT('Origin',(-3.,-1.5334241092205,24.9));
#13215=CARTESIAN_POINT('',(-2.75,-1.5334241092205,24.9));
#13216=CARTESIAN_POINT('',(-3.,-1.5334241092205,24.9));
#13217=CARTESIAN_POINT('',(-2.75,-1.5334241092205,24.9));
#13218=CARTESIAN_POINT('Origin',(-3.,0.625375136733055,24.9));
#13219=CARTESIAN_POINT('',(-2.75,0.625375136733055,24.9));
#13220=CARTESIAN_POINT('',(-3.,0.625375136733055,24.9));
#13221=CARTESIAN_POINT('',(-2.75,0.625375136733055,24.9));
#13222=CARTESIAN_POINT('Origin',(-3.,0.625375136733055,21.7000000715256));
#13223=CARTESIAN_POINT('',(-2.75,0.625375136733055,21.7000000715256));
#13224=CARTESIAN_POINT('Origin',(-2.75,-0.454024486243725,23.3000000357628));
#13225=CARTESIAN_POINT('Ctrl Pts',(-3.90882250993909,1.19290575385094,24.0392854381073));
#13226=CARTESIAN_POINT('Ctrl Pts',(-1.59117749006091,1.19290575385094,24.0392854381073));
#13227=CARTESIAN_POINT('Ctrl Pts',(-3.90882250993909,1.19290575385094,23.6674598658318));
#13228=CARTESIAN_POINT('Ctrl Pts',(-1.59117749006091,1.19290575385094,23.6674598658318));
#13229=CARTESIAN_POINT('Ctrl Pts',(-3.90882250993909,1.19290575385094,23.2956342935562));
#13230=CARTESIAN_POINT('Ctrl Pts',(-1.59117749006091,1.19290575385094,23.2956342935562));
#13231=CARTESIAN_POINT('Ctrl Pts',(-3.90882250993909,1.19290575385094,22.80886759758));
#13232=CARTESIAN_POINT('Ctrl Pts',(-1.59117749006091,1.19290575385094,22.80886759758));
#13233=CARTESIAN_POINT('Ctrl Pts',(-3.90882250993909,1.38935878872872,22.4246930122375));
#13234=CARTESIAN_POINT('Ctrl Pts',(-1.59117749006091,1.38935878872872,22.4246930122375));
#13235=CARTESIAN_POINT('Ctrl Pts',(-3.90882250993909,1.57799645627673,22.0558018024107));
#13236=CARTESIAN_POINT('Ctrl Pts',(-1.59117749006091,1.57799645627673,22.0558018024107));
#13237=CARTESIAN_POINT('Ctrl Pts',(-3.90882250993909,1.76663412382475,21.6869105925839));
#13238=CARTESIAN_POINT('Ctrl Pts',(-1.59117749006091,1.76663412382475,21.6869105925839));
#13239=CARTESIAN_POINT('',(-3.,1.19290575385094,23.2956342935562));
#13240=CARTESIAN_POINT('Ctrl Pts',(-3.,1.37953594326973,24.1545701563358));
#13241=CARTESIAN_POINT('Ctrl Pts',(-2.75,1.37953594326973,24.1545701563358));
#13242=CARTESIAN_POINT('Ctrl Pts',(-3.,1.19290575385094,23.7758526742458));
#13243=CARTESIAN_POINT('Ctrl Pts',(-2.75,1.19290575385094,23.7758526742458));
#13244=CARTESIAN_POINT('Ctrl Pts',(-3.,1.19290575385094,23.2956342935562));
#13245=CARTESIAN_POINT('Ctrl Pts',(-2.75,1.19290575385094,23.2956342935562));
#13246=CARTESIAN_POINT('',(-3.,1.37953594326973,24.1545701563358));
#13247=CARTESIAN_POINT('Ctrl Pts',(-3.,1.92196443676949,24.7450204730034));
#13248=CARTESIAN_POINT('Ctrl Pts',(-2.75,1.92196443676949,24.7450204730034));
#13249=CARTESIAN_POINT('Ctrl Pts',(-3.,1.56616643071175,24.5332877874374));
#13250=CARTESIAN_POINT('Ctrl Pts',(-2.75,1.56616643071175,24.5332877874374));
#13251=CARTESIAN_POINT('Ctrl Pts',(-3.,1.37953594326973,24.1545701563358));
#13252=CARTESIAN_POINT('Ctrl Pts',(-2.75,1.37953594326973,24.1545701563358));
#13253=CARTESIAN_POINT('',(-3.,1.92196443676949,24.7450204730034));
#13254=CARTESIAN_POINT('Ctrl Pts',(-3.,2.72087290883064,24.9567531585693));
#13255=CARTESIAN_POINT('Ctrl Pts',(-2.75,2.72087290883064,24.9567531585693));
#13256=CARTESIAN_POINT('Ctrl Pts',(-3.,2.27776229381562,24.9567531585693));
#13257=CARTESIAN_POINT('Ctrl Pts',(-2.75,2.27776229381562,24.9567531585693));
#13258=CARTESIAN_POINT('Ctrl Pts',(-3.,1.92196443676949,24.7450204730034));
#13259=CARTESIAN_POINT('Ctrl Pts',(-2.75,1.92196443676949,24.7450204730034));
#13260=CARTESIAN_POINT('',(-3.,2.72087290883064,24.9567531585693));
#13261=CARTESIAN_POINT('Ctrl Pts',(-3.,3.82537491619587,24.5060028672218));
#13262=CARTESIAN_POINT('Ctrl Pts',(-2.75,3.82537491619587,24.5060028672218));
#13263=CARTESIAN_POINT('Ctrl Pts',(-3.,3.39754410088063,24.9567531585693));
#13264=CARTESIAN_POINT('Ctrl Pts',(-2.75,3.39754410088063,24.9567531585693));
#13265=CARTESIAN_POINT('Ctrl Pts',(-3.,2.72087290883064,24.9567531585693));
#13266=CARTESIAN_POINT('Ctrl Pts',(-2.75,2.72087290883064,24.9567531585693));
#13267=CARTESIAN_POINT('',(-3.,3.82537491619587,24.5060028672218));
#13268=CARTESIAN_POINT('Ctrl Pts',(-3.,4.25320571288467,23.2585265278816));
#13269=CARTESIAN_POINT('Ctrl Pts',(-2.75,4.25320571288467,23.2585265278816));
#13270=CARTESIAN_POINT('Ctrl Pts',(-3.,4.25320571288467,24.0552522778511));
#13271=CARTESIAN_POINT('Ctrl Pts',(-2.75,4.25320571288467,24.0552522778511));
#13272=CARTESIAN_POINT('Ctrl Pts',(-3.,3.82537491619587,24.5060028672218));
#13273=CARTESIAN_POINT('Ctrl Pts',(-2.75,3.82537491619587,24.5060028672218));
#13274=CARTESIAN_POINT('Origin',(-3.,-4.03055921196938,65.1537516951561));
#13275=CARTESIAN_POINT('',(-2.75,-4.03055921196938,65.1537516951561));
#13276=CARTESIAN_POINT('',(-3.,-4.03055921196938,65.1537516951561));
#13277=CARTESIAN_POINT('',(-2.75,-2.52878561615944,65.1537516951561));
#13278=CARTESIAN_POINT('',(-2.75,-4.03055921196938,65.1537516951561));
#13279=CARTESIAN_POINT('',(-3.,-2.52878561615944,65.1537516951561));
#13280=CARTESIAN_POINT('Origin',(-3.,-4.03055921196938,65.5313779652119));
#13281=CARTESIAN_POINT('',(-2.75,-4.03055921196938,65.5313779652119));
#13282=CARTESIAN_POINT('',(-3.,-4.03055921196938,65.5313779652119));
#13283=CARTESIAN_POINT('',(-2.75,-4.03055921196938,65.5313779652119));
#13284=CARTESIAN_POINT('Origin',(-3.,-2.52878561615944,65.5313779652119));
#13285=CARTESIAN_POINT('',(-2.75,-2.52878561615944,65.5313779652119));
#13286=CARTESIAN_POINT('',(-3.,-2.52878561615944,65.5313779652119));
#13287=CARTESIAN_POINT('',(-2.75,-2.52878561615944,65.5313779652119));
#13288=CARTESIAN_POINT('Origin',(-3.,-2.52878561615944,66.5223738789558));
#13289=CARTESIAN_POINT('',(-2.75,-2.52878561615944,66.5223738789558));
#13290=CARTESIAN_POINT('',(-3.,-2.52878561615944,66.5223738789558));
#13291=CARTESIAN_POINT('',(-2.75,-2.52878561615944,66.5223738789558));
#13292=CARTESIAN_POINT('Origin',(-3.,-4.26411971449852,66.5223738789558));
#13293=CARTESIAN_POINT('',(-2.75,-4.26411971449852,66.5223738789558));
#13294=CARTESIAN_POINT('',(-3.,-4.26411971449852,66.5223738789558));
#13295=CARTESIAN_POINT('',(-2.75,-4.26411971449852,66.5223738789558));
#13296=CARTESIAN_POINT('Origin',(-3.,-4.26411971449852,66.9));
#13297=CARTESIAN_POINT('',(-2.75,-4.26411971449852,66.9));
#13298=CARTESIAN_POINT('',(-3.,-4.26411971449852,66.9));
#13299=CARTESIAN_POINT('',(-2.75,-4.26411971449852,66.9));
#13300=CARTESIAN_POINT('Origin',(-3.,-2.10532046854496,66.9));
#13301=CARTESIAN_POINT('',(-2.75,-2.10532046854496,66.9));
#13302=CARTESIAN_POINT('',(-3.,-2.10532046854496,66.9));
#13303=CARTESIAN_POINT('',(-2.75,-2.10532046854496,66.9));
#13304=CARTESIAN_POINT('Origin',(-3.,-2.10532046854496,63.7000000715256));
#13305=CARTESIAN_POINT('',(-2.75,-2.10532046854496,63.7000000715256));
#13306=CARTESIAN_POINT('',(-3.,-2.10532046854496,63.7000000715256));
#13307=CARTESIAN_POINT('',(-2.75,-2.10532046854496,63.7000000715256));
#13308=CARTESIAN_POINT('Origin',(-3.,-2.52878561615944,63.7000000715256));
#13309=CARTESIAN_POINT('',(-2.75,-2.52878561615944,63.7000000715256));
#13310=CARTESIAN_POINT('',(-3.,-2.52878561615944,63.7000000715256));
#13311=CARTESIAN_POINT('',(-2.75,-2.52878561615944,63.7000000715256));
#13312=CARTESIAN_POINT('Origin',(-3.,-2.52878561615944,65.1537516951561));
#13313=CARTESIAN_POINT('',(-2.75,-2.52878561615944,65.1537516951561));
#13314=CARTESIAN_POINT('Origin',(-2.75,-3.18472009152174,65.3000000357628));
#13315=CARTESIAN_POINT('Origin',(-3.,-1.29986360669136,65.1537516951561));
#13316=CARTESIAN_POINT('',(-2.75,-1.29986360669136,65.1537516951561));
#13317=CARTESIAN_POINT('',(-3.,-1.29986360669136,65.1537516951561));
#13318=CARTESIAN_POINT('',(-2.75,0.201909989118576,65.1537516951561));
#13319=CARTESIAN_POINT('',(-2.75,-1.29986360669136,65.1537516951561));
#13320=CARTESIAN_POINT('',(-3.,0.201909989118576,65.1537516951561));
#13321=CARTESIAN_POINT('Origin',(-3.,-1.29986360669136,65.5313779652119));
#13322=CARTESIAN_POINT('',(-2.75,-1.29986360669136,65.5313779652119));
#13323=CARTESIAN_POINT('',(-3.,-1.29986360669136,65.5313779652119));
#13324=CARTESIAN_POINT('',(-2.75,-1.29986360669136,65.5313779652119));
#13325=CARTESIAN_POINT('Origin',(-3.,0.201909989118576,65.5313779652119));
#13326=CARTESIAN_POINT('',(-2.75,0.201909989118576,65.5313779652119));
#13327=CARTESIAN_POINT('',(-3.,0.201909989118576,65.5313779652119));
#13328=CARTESIAN_POINT('',(-2.75,0.201909989118576,65.5313779652119));
#13329=CARTESIAN_POINT('Origin',(-3.,0.201909989118576,66.5223738789558));
#13330=CARTESIAN_POINT('',(-2.75,0.201909989118576,66.5223738789558));
#13331=CARTESIAN_POINT('',(-3.,0.201909989118576,66.5223738789558));
#13332=CARTESIAN_POINT('',(-2.75,0.201909989118576,66.5223738789558));
#13333=CARTESIAN_POINT('Origin',(-3.,-1.5334241092205,66.5223738789558));
#13334=CARTESIAN_POINT('',(-2.75,-1.5334241092205,66.5223738789558));
#13335=CARTESIAN_POINT('',(-3.,-1.5334241092205,66.5223738789558));
#13336=CARTESIAN_POINT('',(-2.75,-1.5334241092205,66.5223738789558));
#13337=CARTESIAN_POINT('Origin',(-3.,-1.5334241092205,66.9));
#13338=CARTESIAN_POINT('',(-2.75,-1.5334241092205,66.9));
#13339=CARTESIAN_POINT('',(-3.,-1.5334241092205,66.9));
#13340=CARTESIAN_POINT('',(-2.75,-1.5334241092205,66.9));
#13341=CARTESIAN_POINT('Origin',(-3.,0.625375136733055,66.9));
#13342=CARTESIAN_POINT('',(-2.75,0.625375136733055,66.9));
#13343=CARTESIAN_POINT('',(-3.,0.625375136733055,66.9));
#13344=CARTESIAN_POINT('',(-2.75,0.625375136733055,66.9));
#13345=CARTESIAN_POINT('Origin',(-3.,0.625375136733055,63.7000000715256));
#13346=CARTESIAN_POINT('',(-2.75,0.625375136733055,63.7000000715256));
#13347=CARTESIAN_POINT('',(-3.,0.625375136733055,63.7000000715256));
#13348=CARTESIAN_POINT('',(-2.75,0.625375136733055,63.7000000715256));
#13349=CARTESIAN_POINT('Origin',(-3.,0.201909989118576,63.7000000715256));
#13350=CARTESIAN_POINT('',(-2.75,0.201909989118576,63.7000000715256));
#13351=CARTESIAN_POINT('',(-3.,0.201909989118576,63.7000000715256));
#13352=CARTESIAN_POINT('',(-2.75,0.201909989118576,63.7000000715256));
#13353=CARTESIAN_POINT('Origin',(-3.,0.201909989118576,65.1537516951561));
#13354=CARTESIAN_POINT('',(-2.75,0.201909989118576,65.1537516951561));
#13355=CARTESIAN_POINT('Origin',(-2.75,-0.454024486243725,65.3000000357628));
#13356=CARTESIAN_POINT('Ctrl Pts',(-3.,2.72305563092232,63.6454299330711));
#13357=CARTESIAN_POINT('Ctrl Pts',(-2.75,2.72305563092232,63.6454299330711));
#13358=CARTESIAN_POINT('Ctrl Pts',(-3.,3.17489743232727,63.6454299330711));
#13359=CARTESIAN_POINT('Ctrl Pts',(-2.75,3.17489743232727,63.6454299330711));
#13360=CARTESIAN_POINT('Ctrl Pts',(-3.,3.53069551289082,63.8637107849121));
#13361=CARTESIAN_POINT('Ctrl Pts',(-2.75,3.53069551289082,63.8637107849121));
#13362=CARTESIAN_POINT('',(-2.75,2.72305563092232,63.6454299330711));
#13363=CARTESIAN_POINT('',(-3.,2.72305563092232,63.6454299330711));
#13364=CARTESIAN_POINT('',(-2.75,3.53069551289082,63.8637107849121));
#13365=CARTESIAN_POINT('Ctrl Pts',(-2.75,2.72305563092232,63.6454299330711));
#13366=CARTESIAN_POINT('Ctrl Pts',(-2.75,3.17489743232727,63.6454299330711));
#13367=CARTESIAN_POINT('Ctrl Pts',(-2.75,3.53069551289082,63.8637107849121));
#13368=CARTESIAN_POINT('',(-3.,3.53069551289082,63.8637107849121));
#13369=CARTESIAN_POINT('Ctrl Pts',(-3.,1.94597527384758,63.8429740309715));
#13370=CARTESIAN_POINT('Ctrl Pts',(-2.75,1.94597527384758,63.8429740309715));
#13371=CARTESIAN_POINT('Ctrl Pts',(-3.,2.30613887310028,63.6454299330711));
#13372=CARTESIAN_POINT('Ctrl Pts',(-2.75,2.30613887310028,63.6454299330711));
#13373=CARTESIAN_POINT('Ctrl Pts',(-3.,2.72305563092232,63.6454299330711));
#13374=CARTESIAN_POINT('Ctrl Pts',(-2.75,2.72305563092232,63.6454299330711));
#13375=CARTESIAN_POINT('',(-2.75,1.94597527384758,63.8429740309715));
#13376=CARTESIAN_POINT('',(-3.,1.94597527384758,63.8429740309715));
#13377=CARTESIAN_POINT('Ctrl Pts',(-2.75,1.94597527384758,63.8429740309715));
#13378=CARTESIAN_POINT('Ctrl Pts',(-2.75,2.30613887310028,63.6454299330711));
#13379=CARTESIAN_POINT('Ctrl Pts',(-2.75,2.72305563092232,63.6454299330711));
#13380=CARTESIAN_POINT('Ctrl Pts',(-3.,1.38935878872872,64.4246930122376));
#13381=CARTESIAN_POINT('Ctrl Pts',(-2.75,1.38935878872872,64.4246930122376));
#13382=CARTESIAN_POINT('Ctrl Pts',(-3.,1.58581152558327,64.0405184268951));
#13383=CARTESIAN_POINT('Ctrl Pts',(-2.75,1.58581152558327,64.0405184268951));
#13384=CARTESIAN_POINT('Ctrl Pts',(-3.,1.94597527384758,63.8429740309715));
#13385=CARTESIAN_POINT('Ctrl Pts',(-2.75,1.94597527384758,63.8429740309715));
#13386=CARTESIAN_POINT('',(-2.75,1.38935878872872,64.4246930122376));
#13387=CARTESIAN_POINT('',(-3.,1.38935878872872,64.4246930122376));
#13388=CARTESIAN_POINT('Ctrl Pts',(-2.75,1.38935878872872,64.4246930122376));
#13389=CARTESIAN_POINT('Ctrl Pts',(-2.75,1.58581152558327,64.0405184268951));
#13390=CARTESIAN_POINT('Ctrl Pts',(-2.75,1.94597527384758,63.8429740309715));
#13391=CARTESIAN_POINT('Ctrl Pts',(-3.,1.19290575385094,65.2956342935562));
#13392=CARTESIAN_POINT('Ctrl Pts',(-2.75,1.19290575385094,65.2956342935562));
#13393=CARTESIAN_POINT('Ctrl Pts',(-3.,1.19290575385094,64.80886759758));
#13394=CARTESIAN_POINT('Ctrl Pts',(-2.75,1.19290575385094,64.80886759758));
#13395=CARTESIAN_POINT('Ctrl Pts',(-3.,1.38935878872872,64.4246930122376));
#13396=CARTESIAN_POINT('Ctrl Pts',(-2.75,1.38935878872872,64.4246930122376));
#13397=CARTESIAN_POINT('',(-2.75,1.19290575385094,65.2956342935562));
#13398=CARTESIAN_POINT('',(-3.,1.19290575385094,65.2956342935562));
#13399=CARTESIAN_POINT('Ctrl Pts',(-2.75,1.19290575385094,65.2956342935562));
#13400=CARTESIAN_POINT('Ctrl Pts',(-2.75,1.19290575385094,64.80886759758));
#13401=CARTESIAN_POINT('Ctrl Pts',(-2.75,1.38935878872872,64.4246930122376));
#13402=CARTESIAN_POINT('Ctrl Pts',(-3.,1.37953594326973,66.1545701563358));
#13403=CARTESIAN_POINT('Ctrl Pts',(-2.75,1.37953594326973,66.1545701563358));
#13404=CARTESIAN_POINT('Ctrl Pts',(-3.,1.19290575385094,65.7758526742458));
#13405=CARTESIAN_POINT('Ctrl Pts',(-2.75,1.19290575385094,65.7758526742458));
#13406=CARTESIAN_POINT('Ctrl Pts',(-3.,1.19290575385094,65.2956342935562));
#13407=CARTESIAN_POINT('Ctrl Pts',(-2.75,1.19290575385094,65.2956342935562));
#13408=CARTESIAN_POINT('',(-2.75,1.37953594326973,66.1545701563358));
#13409=CARTESIAN_POINT('',(-3.,1.37953594326973,66.1545701563358));
#13410=CARTESIAN_POINT('Ctrl Pts',(-2.75,1.37953594326973,66.1545701563358));
#13411=CARTESIAN_POINT('Ctrl Pts',(-2.75,1.19290575385094,65.7758526742458));
#13412=CARTESIAN_POINT('Ctrl Pts',(-2.75,1.19290575385094,65.2956342935562));
#13413=CARTESIAN_POINT('Ctrl Pts',(-3.,1.92196443676949,66.7450204730034));
#13414=CARTESIAN_POINT('Ctrl Pts',(-2.75,1.92196443676949,66.7450204730034));
#13415=CARTESIAN_POINT('Ctrl Pts',(-3.,1.56616643071175,66.5332877874374));
#13416=CARTESIAN_POINT('Ctrl Pts',(-2.75,1.56616643071175,66.5332877874374));
#13417=CARTESIAN_POINT('Ctrl Pts',(-3.,1.37953594326973,66.1545701563358));
#13418=CARTESIAN_POINT('Ctrl Pts',(-2.75,1.37953594326973,66.1545701563358));
#13419=CARTESIAN_POINT('',(-2.75,1.92196443676949,66.7450204730034));
#13420=CARTESIAN_POINT('',(-3.,1.92196443676949,66.7450204730034));
#13421=CARTESIAN_POINT('Ctrl Pts',(-2.75,1.92196443676949,66.7450204730034));
#13422=CARTESIAN_POINT('Ctrl Pts',(-2.75,1.56616643071175,66.5332877874374));
#13423=CARTESIAN_POINT('Ctrl Pts',(-2.75,1.37953594326973,66.1545701563358));
#13424=CARTESIAN_POINT('Ctrl Pts',(-3.,2.72087290883064,66.9567531585693));
#13425=CARTESIAN_POINT('Ctrl Pts',(-2.75,2.72087290883064,66.9567531585693));
#13426=CARTESIAN_POINT('Ctrl Pts',(-3.,2.27776229381562,66.9567531585693));
#13427=CARTESIAN_POINT('Ctrl Pts',(-2.75,2.27776229381562,66.9567531585693));
#13428=CARTESIAN_POINT('Ctrl Pts',(-3.,1.92196443676949,66.7450204730034));
#13429=CARTESIAN_POINT('Ctrl Pts',(-2.75,1.92196443676949,66.7450204730034));
#13430=CARTESIAN_POINT('',(-2.75,2.72087290883064,66.9567531585693));
#13431=CARTESIAN_POINT('',(-3.,2.72087290883064,66.9567531585693));
#13432=CARTESIAN_POINT('Ctrl Pts',(-2.75,2.72087290883064,66.9567531585693));
#13433=CARTESIAN_POINT('Ctrl Pts',(-2.75,2.27776229381562,66.9567531585693));
#13434=CARTESIAN_POINT('Ctrl Pts',(-2.75,1.92196443676949,66.7450204730034));
#13435=CARTESIAN_POINT('Ctrl Pts',(-3.,3.82537491619587,66.5060028672218));
#13436=CARTESIAN_POINT('Ctrl Pts',(-2.75,3.82537491619587,66.5060028672218));
#13437=CARTESIAN_POINT('Ctrl Pts',(-3.,3.39754410088063,66.9567531585693));
#13438=CARTESIAN_POINT('Ctrl Pts',(-2.75,3.39754410088063,66.9567531585693));
#13439=CARTESIAN_POINT('Ctrl Pts',(-3.,2.72087290883064,66.9567531585693));
#13440=CARTESIAN_POINT('Ctrl Pts',(-2.75,2.72087290883064,66.9567531585693));
#13441=CARTESIAN_POINT('',(-2.75,3.82537491619587,66.5060028672218));
#13442=CARTESIAN_POINT('',(-3.,3.82537491619587,66.5060028672218));
#13443=CARTESIAN_POINT('Ctrl Pts',(-2.75,3.82537491619587,66.5060028672218));
#13444=CARTESIAN_POINT('Ctrl Pts',(-2.75,3.39754410088063,66.9567531585693));
#13445=CARTESIAN_POINT('Ctrl Pts',(-2.75,2.72087290883064,66.9567531585693));
#13446=CARTESIAN_POINT('Ctrl Pts',(-3.,4.25320571288467,65.2585265278816));
#13447=CARTESIAN_POINT('Ctrl Pts',(-2.75,4.25320571288467,65.2585265278816));
#13448=CARTESIAN_POINT('Ctrl Pts',(-3.,4.25320571288467,66.0552522778511));
#13449=CARTESIAN_POINT('Ctrl Pts',(-2.75,4.25320571288467,66.0552522778511));
#13450=CARTESIAN_POINT('Ctrl Pts',(-3.,3.82537491619587,66.5060028672218));
#13451=CARTESIAN_POINT('Ctrl Pts',(-2.75,3.82537491619587,66.5060028672218));
#13452=CARTESIAN_POINT('',(-2.75,4.25320571288467,65.2585265278816));
#13453=CARTESIAN_POINT('',(-3.,4.25320571288467,65.2585265278816));
#13454=CARTESIAN_POINT('Ctrl Pts',(-2.75,4.25320571288467,65.2585265278816));
#13455=CARTESIAN_POINT('Ctrl Pts',(-2.75,4.25320571288467,66.0552522778511));
#13456=CARTESIAN_POINT('Ctrl Pts',(-2.75,3.82537491619587,66.5060028672218));
#13457=CARTESIAN_POINT('Ctrl Pts',(-3.,4.06984962522984,64.4596180558205));
#13458=CARTESIAN_POINT('Ctrl Pts',(-2.75,4.06984962522984,64.4596180558205));
#13459=CARTESIAN_POINT('Ctrl Pts',(-3.,4.25320571288467,64.8372441768646));
#13460=CARTESIAN_POINT('Ctrl Pts',(-2.75,4.25320571288467,64.8372441768646));
#13461=CARTESIAN_POINT('Ctrl Pts',(-3.,4.25320571288467,65.2585265278816));
#13462=CARTESIAN_POINT('Ctrl Pts',(-2.75,4.25320571288467,65.2585265278816));
#13463=CARTESIAN_POINT('',(-2.75,4.06984962522984,64.4596180558205));
#13464=CARTESIAN_POINT('',(-3.,4.06984962522984,64.4596180558205));
#13465=CARTESIAN_POINT('Ctrl Pts',(-2.75,4.06984962522984,64.4596180558205));
#13466=CARTESIAN_POINT('Ctrl Pts',(-2.75,4.25320571288467,64.8372441768646));
#13467=CARTESIAN_POINT('Ctrl Pts',(-2.75,4.25320571288467,65.2585265278816));
#13468=CARTESIAN_POINT('Ctrl Pts',(-3.,3.53069551289082,63.8637107849121));
#13469=CARTESIAN_POINT('Ctrl Pts',(-2.75,3.53069551289082,63.8637107849121));
#13470=CARTESIAN_POINT('Ctrl Pts',(-3.,3.88649359345436,64.0819919347763));
#13471=CARTESIAN_POINT('Ctrl Pts',(-2.75,3.88649359345436,64.0819919347763));
#13472=CARTESIAN_POINT('Ctrl Pts',(-3.,4.06984962522984,64.4596180558205));
#13473=CARTESIAN_POINT('Ctrl Pts',(-2.75,4.06984962522984,64.4596180558205));
#13474=CARTESIAN_POINT('Ctrl Pts',(-2.75,3.53069551289082,63.8637107849121));
#13475=CARTESIAN_POINT('Ctrl Pts',(-2.75,3.88649359345436,64.0819919347763));
#13476=CARTESIAN_POINT('Ctrl Pts',(-2.75,4.06984962522984,64.4596180558205));
#13477=CARTESIAN_POINT('Origin',(-2.75,2.7230557333678,65.3010915458202));
#13478=CARTESIAN_POINT('Origin',(-3.,16.3103681504726,41.4999999403954));
#13479=CARTESIAN_POINT('',(-2.75,16.3103681504726,41.4999999403954));
#13480=CARTESIAN_POINT('',(-3.,16.3103681504726,41.4999999403954));
#13481=CARTESIAN_POINT('',(-2.75,18.4113232493401,44.6432467103004));
#13482=CARTESIAN_POINT('',(-2.75,16.3103681504726,41.4999999403954));
#13483=CARTESIAN_POINT('',(-3.,18.4113232493401,44.6432467103004));
#13484=CARTESIAN_POINT('Origin',(-3.,15.7673942744732,41.4999999403954));
#13485=CARTESIAN_POINT('',(-2.75,15.7673942744732,41.4999999403954));
#13486=CARTESIAN_POINT('',(-3.,15.7673942744732,41.4999999403954));
#13487=CARTESIAN_POINT('',(-2.75,15.7673942744732,41.4999999403954));
#13488=CARTESIAN_POINT('Origin',(-3.,15.7673942744732,45.5));
#13489=CARTESIAN_POINT('',(-2.75,15.7673942744732,45.5));
#13490=CARTESIAN_POINT('',(-3.,15.7673942744732,45.5));
#13491=CARTESIAN_POINT('',(-2.75,15.7673942744732,45.5));
#13492=CARTESIAN_POINT('Origin',(-3.,16.2748974263668,45.5));
#13493=CARTESIAN_POINT('',(-2.75,16.2748974263668,45.5));
#13494=CARTESIAN_POINT('',(-3.,16.2748974263668,45.5));
#13495=CARTESIAN_POINT('',(-2.75,16.2748974263668,45.5));
#13496=CARTESIAN_POINT('Origin',(-3.,16.2748974263668,42.3594816327095));
#13497=CARTESIAN_POINT('',(-2.75,16.2748974263668,42.3594816327095));
#13498=CARTESIAN_POINT('',(-3.,16.2748974263668,42.3594816327095));
#13499=CARTESIAN_POINT('',(-2.75,16.2748974263668,42.3594816327095));
#13500=CARTESIAN_POINT('Origin',(-3.,18.3758525252342,45.5));
#13501=CARTESIAN_POINT('',(-2.75,18.3758525252342,45.5));
#13502=CARTESIAN_POINT('',(-3.,18.3758525252342,45.5));
#13503=CARTESIAN_POINT('',(-2.75,18.3758525252342,45.5));
#13504=CARTESIAN_POINT('Origin',(-3.,18.9188266247511,45.5));
#13505=CARTESIAN_POINT('',(-2.75,18.9188266247511,45.5));
#13506=CARTESIAN_POINT('',(-3.,18.9188266247511,45.5));
#13507=CARTESIAN_POINT('',(-2.75,18.9188266247511,45.5));
#13508=CARTESIAN_POINT('Origin',(-3.,18.9188266247511,41.4999999403954));
#13509=CARTESIAN_POINT('',(-2.75,18.9188266247511,41.4999999403954));
#13510=CARTESIAN_POINT('',(-3.,18.9188266247511,41.4999999403954));
#13511=CARTESIAN_POINT('',(-2.75,18.9188266247511,41.4999999403954));
#13512=CARTESIAN_POINT('Origin',(-3.,18.4113232493401,41.4999999403954));
#13513=CARTESIAN_POINT('',(-2.75,18.4113232493401,41.4999999403954));
#13514=CARTESIAN_POINT('',(-3.,18.4113232493401,41.4999999403954));
#13515=CARTESIAN_POINT('',(-2.75,18.4113232493401,41.4999999403954));
#13516=CARTESIAN_POINT('Origin',(-3.,18.4113232493401,44.6432467103004));
#13517=CARTESIAN_POINT('',(-2.75,18.4113232493401,44.6432467103004));
#13518=CARTESIAN_POINT('Origin',(-2.75,17.3431104496121,43.4999999701977));
#13519=CARTESIAN_POINT('Ctrl Pts',(-3.,21.5081855356693,41.4317871928215));
#13520=CARTESIAN_POINT('Ctrl Pts',(-2.75,21.5081855356693,41.4317871928215));
#13521=CARTESIAN_POINT('Ctrl Pts',(-3.,22.0729876756668,41.4317871928215));
#13522=CARTESIAN_POINT('Ctrl Pts',(-2.75,22.0729876756668,41.4317871928215));
#13523=CARTESIAN_POINT('Ctrl Pts',(-3.,22.5177353322506,41.7046384811401));
#13524=CARTESIAN_POINT('Ctrl Pts',(-2.75,22.5177353322506,41.7046384811401));
#13525=CARTESIAN_POINT('',(-2.75,21.5081855356693,41.4317871928215));
#13526=CARTESIAN_POINT('',(-3.,21.5081855356693,41.4317871928215));
#13527=CARTESIAN_POINT('',(-2.75,22.5177353322506,41.7046384811401));
#13528=CARTESIAN_POINT('Ctrl Pts',(-2.75,21.5081855356693,41.4317871928215));
#13529=CARTESIAN_POINT('Ctrl Pts',(-2.75,22.0729876756668,41.4317871928215));
#13530=CARTESIAN_POINT('Ctrl Pts',(-2.75,22.5177353322506,41.7046384811401));
#13531=CARTESIAN_POINT('',(-3.,22.5177353322506,41.7046384811401));
#13532=CARTESIAN_POINT('Ctrl Pts',(-3.,20.5368348658085,41.6787176132202));
#13533=CARTESIAN_POINT('Ctrl Pts',(-2.75,20.5368348658085,41.6787176132202));
#13534=CARTESIAN_POINT('Ctrl Pts',(-3.,20.9870394766331,41.4317871928215));
#13535=CARTESIAN_POINT('Ctrl Pts',(-2.75,20.9870394766331,41.4317871928215));
#13536=CARTESIAN_POINT('Ctrl Pts',(-3.,21.5081855356693,41.4317871928215));
#13537=CARTESIAN_POINT('Ctrl Pts',(-2.75,21.5081855356693,41.4317871928215));
#13538=CARTESIAN_POINT('',(-2.75,20.5368348658085,41.6787176132202));
#13539=CARTESIAN_POINT('',(-3.,20.5368348658085,41.6787176132202));
#13540=CARTESIAN_POINT('Ctrl Pts',(-2.75,20.5368348658085,41.6787176132202));
#13541=CARTESIAN_POINT('Ctrl Pts',(-2.75,20.9870394766331,41.4317871928215));
#13542=CARTESIAN_POINT('Ctrl Pts',(-2.75,21.5081855356693,41.4317871928215));
#13543=CARTESIAN_POINT('Ctrl Pts',(-3.,19.8410638868809,42.4058662652969));
#13544=CARTESIAN_POINT('Ctrl Pts',(-2.75,19.8410638868809,42.4058662652969));
#13545=CARTESIAN_POINT('Ctrl Pts',(-3.,20.0866302549839,41.9256480336189));
#13546=CARTESIAN_POINT('Ctrl Pts',(-2.75,20.0866302549839,41.9256480336189));
#13547=CARTESIAN_POINT('Ctrl Pts',(-3.,20.5368348658085,41.6787176132202));
#13548=CARTESIAN_POINT('Ctrl Pts',(-2.75,20.5368348658085,41.6787176132202));
#13549=CARTESIAN_POINT('',(-2.75,19.8410638868809,42.4058662652969));
#13550=CARTESIAN_POINT('',(-3.,19.8410638868809,42.4058662652969));
#13551=CARTESIAN_POINT('Ctrl Pts',(-2.75,19.8410638868809,42.4058662652969));
#13552=CARTESIAN_POINT('Ctrl Pts',(-2.75,20.0866302549839,41.9256480336189));
#13553=CARTESIAN_POINT('Ctrl Pts',(-2.75,20.5368348658085,41.6787176132202));
#13554=CARTESIAN_POINT('Ctrl Pts',(-3.,19.5954978168011,43.4945430159569));
#13555=CARTESIAN_POINT('Ctrl Pts',(-2.75,19.5954978168011,43.4945430159569));
#13556=CARTESIAN_POINT('Ctrl Pts',(-3.,19.5954978168011,42.8860844969749));
#13557=CARTESIAN_POINT('Ctrl Pts',(-2.75,19.5954978168011,42.8860844969749));
#13558=CARTESIAN_POINT('Ctrl Pts',(-3.,19.8410638868809,42.4058662652969));
#13559=CARTESIAN_POINT('Ctrl Pts',(-2.75,19.8410638868809,42.4058662652969));
#13560=CARTESIAN_POINT('',(-2.75,19.5954978168011,43.4945430159569));
#13561=CARTESIAN_POINT('',(-3.,19.5954978168011,43.4945430159569));
#13562=CARTESIAN_POINT('Ctrl Pts',(-2.75,19.5954978168011,43.4945430159569));
#13563=CARTESIAN_POINT('Ctrl Pts',(-2.75,19.5954978168011,42.8860844969749));
#13564=CARTESIAN_POINT('Ctrl Pts',(-2.75,19.8410638868809,42.4058662652969));
#13565=CARTESIAN_POINT('Ctrl Pts',(-3.,19.8287856280804,44.5682128071785));
#13566=CARTESIAN_POINT('Ctrl Pts',(-2.75,19.8287856280804,44.5682128071785));
#13567=CARTESIAN_POINT('Ctrl Pts',(-3.,19.5954978168011,44.0948157310486));
#13568=CARTESIAN_POINT('Ctrl Pts',(-2.75,19.5954978168011,44.0948157310486));
#13569=CARTESIAN_POINT('Ctrl Pts',(-3.,19.5954978168011,43.4945430159569));
#13570=CARTESIAN_POINT('Ctrl Pts',(-2.75,19.5954978168011,43.4945430159569));
#13571=CARTESIAN_POINT('',(-2.75,19.8287856280804,44.5682128071785));
#13572=CARTESIAN_POINT('',(-3.,19.8287856280804,44.5682128071785));
#13573=CARTESIAN_POINT('Ctrl Pts',(-2.75,19.8287856280804,44.5682128071785));
#13574=CARTESIAN_POINT('Ctrl Pts',(-2.75,19.5954978168011,44.0948157310486));
#13575=CARTESIAN_POINT('Ctrl Pts',(-2.75,19.5954978168011,43.4945430159569));
#13576=CARTESIAN_POINT('Ctrl Pts',(-3.,20.5068212449551,45.30627566576));
#13577=CARTESIAN_POINT('Ctrl Pts',(-2.75,20.5068212449551,45.30627566576));
#13578=CARTESIAN_POINT('Ctrl Pts',(-3.,20.0620734393597,45.0416098833084));
#13579=CARTESIAN_POINT('Ctrl Pts',(-2.75,20.0620734393597,45.0416098833084));
#13580=CARTESIAN_POINT('Ctrl Pts',(-3.,19.8287856280804,44.5682128071785));
#13581=CARTESIAN_POINT('Ctrl Pts',(-2.75,19.8287856280804,44.5682128071785));
#13582=CARTESIAN_POINT('',(-2.75,20.5068212449551,45.30627566576));
#13583=CARTESIAN_POINT('',(-3.,20.5068212449551,45.30627566576));
#13584=CARTESIAN_POINT('Ctrl Pts',(-2.75,20.5068212449551,45.30627566576));
#13585=CARTESIAN_POINT('Ctrl Pts',(-2.75,20.0620734393597,45.0416098833084));
#13586=CARTESIAN_POINT('Ctrl Pts',(-2.75,19.8287856280804,44.5682128071785));
#13587=CARTESIAN_POINT('Ctrl Pts',(-3.,21.5054569840431,45.5709411501884));
#13588=CARTESIAN_POINT('Ctrl Pts',(-2.75,21.5054569840431,45.5709411501884));
#13589=CARTESIAN_POINT('Ctrl Pts',(-3.,20.9515687525272,45.5709411501884));
#13590=CARTESIAN_POINT('Ctrl Pts',(-2.75,20.9515687525272,45.5709411501884));
#13591=CARTESIAN_POINT('Ctrl Pts',(-3.,20.5068212449551,45.30627566576));
#13592=CARTESIAN_POINT('Ctrl Pts',(-2.75,20.5068212449551,45.30627566576));
#13593=CARTESIAN_POINT('',(-2.75,21.5054569840431,45.5709411501884));
#13594=CARTESIAN_POINT('',(-3.,21.5054569840431,45.5709411501884));
#13595=CARTESIAN_POINT('Ctrl Pts',(-2.75,21.5054569840431,45.5709411501884));
#13596=CARTESIAN_POINT('Ctrl Pts',(-2.75,20.9515687525272,45.5709411501884));
#13597=CARTESIAN_POINT('Ctrl Pts',(-2.75,20.5068212449551,45.30627566576));
#13598=CARTESIAN_POINT('Ctrl Pts',(-3.,22.8860845863819,45.0075035095215));
#13599=CARTESIAN_POINT('Ctrl Pts',(-2.75,22.8860845863819,45.0075035095215));
#13600=CARTESIAN_POINT('Ctrl Pts',(-3.,22.3512960672379,45.5709411501884));
#13601=CARTESIAN_POINT('Ctrl Pts',(-2.75,22.3512960672379,45.5709411501884));
#13602=CARTESIAN_POINT('Ctrl Pts',(-3.,21.5054569840431,45.5709411501884));
#13603=CARTESIAN_POINT('Ctrl Pts',(-2.75,21.5054569840431,45.5709411501884));
#13604=CARTESIAN_POINT('',(-2.75,22.8860845863819,45.0075035095215));
#13605=CARTESIAN_POINT('',(-3.,22.8860845863819,45.0075035095215));
#13606=CARTESIAN_POINT('Ctrl Pts',(-2.75,22.8860845863819,45.0075035095215));
#13607=CARTESIAN_POINT('Ctrl Pts',(-2.75,22.3512960672379,45.5709411501884));
#13608=CARTESIAN_POINT('Ctrl Pts',(-2.75,21.5054569840431,45.5709411501884));
#13609=CARTESIAN_POINT('Ctrl Pts',(-3.,23.4208730682731,43.4481580853462));
#13610=CARTESIAN_POINT('Ctrl Pts',(-2.75,23.4208730682731,43.4481580853462));
#13611=CARTESIAN_POINT('Ctrl Pts',(-3.,23.4208730682731,44.4440655708313));
#13612=CARTESIAN_POINT('Ctrl Pts',(-2.75,23.4208730682731,44.4440655708313));
#13613=CARTESIAN_POINT('Ctrl Pts',(-3.,22.8860845863819,45.0075035095215));
#13614=CARTESIAN_POINT('Ctrl Pts',(-2.75,22.8860845863819,45.0075035095215));
#13615=CARTESIAN_POINT('',(-2.75,23.4208730682731,43.4481580853462));
#13616=CARTESIAN_POINT('',(-3.,23.4208730682731,43.4481580853462));
#13617=CARTESIAN_POINT('Ctrl Pts',(-2.75,23.4208730682731,43.4481580853462));
#13618=CARTESIAN_POINT('Ctrl Pts',(-2.75,23.4208730682731,44.4440655708313));
#13619=CARTESIAN_POINT('Ctrl Pts',(-2.75,22.8860845863819,45.0075035095215));
#13620=CARTESIAN_POINT('Ctrl Pts',(-3.,23.1916779726744,42.4495224952698));
#13621=CARTESIAN_POINT('Ctrl Pts',(-2.75,23.1916779726744,42.4495224952698));
#13622=CARTESIAN_POINT('Ctrl Pts',(-3.,23.4208730682731,42.9215552210808));
#13623=CARTESIAN_POINT('Ctrl Pts',(-2.75,23.4208730682731,42.9215552210808));
#13624=CARTESIAN_POINT('Ctrl Pts',(-3.,23.4208730682731,43.4481580853462));
#13625=CARTESIAN_POINT('Ctrl Pts',(-2.75,23.4208730682731,43.4481580853462));
#13626=CARTESIAN_POINT('',(-2.75,23.1916779726744,42.4495224952698));
#13627=CARTESIAN_POINT('',(-3.,23.1916779726744,42.4495224952698));
#13628=CARTESIAN_POINT('Ctrl Pts',(-2.75,23.1916779726744,42.4495224952698));
#13629=CARTESIAN_POINT('Ctrl Pts',(-2.75,23.4208730682731,42.9215552210808));
#13630=CARTESIAN_POINT('Ctrl Pts',(-2.75,23.4208730682731,43.4481580853462));
#13631=CARTESIAN_POINT('Ctrl Pts',(-3.,22.5177353322506,41.7046384811401));
#13632=CARTESIAN_POINT('Ctrl Pts',(-2.75,22.5177353322506,41.7046384811401));
#13633=CARTESIAN_POINT('Ctrl Pts',(-3.,22.9624829143286,41.9774897694588));
#13634=CARTESIAN_POINT('Ctrl Pts',(-2.75,22.9624829143286,41.9774897694588));
#13635=CARTESIAN_POINT('Ctrl Pts',(-3.,23.1916779726744,42.4495224952698));
#13636=CARTESIAN_POINT('Ctrl Pts',(-2.75,23.1916779726744,42.4495224952698));
#13637=CARTESIAN_POINT('Ctrl Pts',(-2.75,22.5177353322506,41.7046384811401));
#13638=CARTESIAN_POINT('Ctrl Pts',(-2.75,22.9624829143286,41.9774897694588));
#13639=CARTESIAN_POINT('Ctrl Pts',(-2.75,23.1916779726744,42.4495224952698));
#13640=CARTESIAN_POINT('Origin',(-2.75,21.5081854425371,43.501364171505));
#13641=CARTESIAN_POINT('Origin',(-3.,-22.6896318495274,41.4999999403954));
#13642=CARTESIAN_POINT('',(-2.75,-22.6896318495274,41.4999999403954));
#13643=CARTESIAN_POINT('',(-3.,-22.6896318495274,41.4999999403954));
#13644=CARTESIAN_POINT('',(-2.75,-20.5886767506599,44.6432467103004));
#13645=CARTESIAN_POINT('',(-2.75,-22.6896318495274,41.4999999403954));
#13646=CARTESIAN_POINT('',(-3.,-20.5886767506599,44.6432467103004));
#13647=CARTESIAN_POINT('Origin',(-3.,-23.2326057255268,41.4999999403954));
#13648=CARTESIAN_POINT('',(-2.75,-23.2326057255268,41.4999999403954));
#13649=CARTESIAN_POINT('',(-3.,-23.2326057255268,41.4999999403954));
#13650=CARTESIAN_POINT('',(-2.75,-23.2326057255268,41.4999999403954));
#13651=CARTESIAN_POINT('Origin',(-3.,-23.2326057255268,45.5));
#13652=CARTESIAN_POINT('',(-2.75,-23.2326057255268,45.5));
#13653=CARTESIAN_POINT('',(-3.,-23.2326057255268,45.5));
#13654=CARTESIAN_POINT('',(-2.75,-23.2326057255268,45.5));
#13655=CARTESIAN_POINT('Origin',(-3.,-22.7251025736332,45.5));
#13656=CARTESIAN_POINT('',(-2.75,-22.7251025736332,45.5));
#13657=CARTESIAN_POINT('',(-3.,-22.7251025736332,45.5));
#13658=CARTESIAN_POINT('',(-2.75,-22.7251025736332,45.5));
#13659=CARTESIAN_POINT('Origin',(-3.,-22.7251025736332,42.3594816327095));
#13660=CARTESIAN_POINT('',(-2.75,-22.7251025736332,42.3594816327095));
#13661=CARTESIAN_POINT('',(-3.,-22.7251025736332,42.3594816327095));
#13662=CARTESIAN_POINT('',(-2.75,-22.7251025736332,42.3594816327095));
#13663=CARTESIAN_POINT('Origin',(-3.,-20.6241474747658,45.5));
#13664=CARTESIAN_POINT('',(-2.75,-20.6241474747658,45.5));
#13665=CARTESIAN_POINT('',(-3.,-20.6241474747658,45.5));
#13666=CARTESIAN_POINT('',(-2.75,-20.6241474747658,45.5));
#13667=CARTESIAN_POINT('Origin',(-3.,-20.0811733752489,45.5));
#13668=CARTESIAN_POINT('',(-2.75,-20.0811733752489,45.5));
#13669=CARTESIAN_POINT('',(-3.,-20.0811733752489,45.5));
#13670=CARTESIAN_POINT('',(-2.75,-20.0811733752489,45.5));
#13671=CARTESIAN_POINT('Origin',(-3.,-20.0811733752489,41.4999999403954));
#13672=CARTESIAN_POINT('',(-2.75,-20.0811733752489,41.4999999403954));
#13673=CARTESIAN_POINT('',(-3.,-20.0811733752489,41.4999999403954));
#13674=CARTESIAN_POINT('',(-2.75,-20.0811733752489,41.4999999403954));
#13675=CARTESIAN_POINT('Origin',(-3.,-20.5886767506599,41.4999999403954));
#13676=CARTESIAN_POINT('',(-2.75,-20.5886767506599,41.4999999403954));
#13677=CARTESIAN_POINT('',(-3.,-20.5886767506599,41.4999999403954));
#13678=CARTESIAN_POINT('',(-2.75,-20.5886767506599,41.4999999403954));
#13679=CARTESIAN_POINT('Origin',(-3.,-20.5886767506599,44.6432467103004));
#13680=CARTESIAN_POINT('',(-2.75,-20.5886767506599,44.6432467103004));
#13681=CARTESIAN_POINT('Origin',(-2.75,-21.6568895503879,43.4999999701977));
#13682=CARTESIAN_POINT('Ctrl Pts',(-3.,-17.4918144643307,41.4317871928215));
#13683=CARTESIAN_POINT('Ctrl Pts',(-2.75,-17.4918144643307,41.4317871928215));
#13684=CARTESIAN_POINT('Ctrl Pts',(-3.,-16.9270123243332,41.4317871928215));
#13685=CARTESIAN_POINT('Ctrl Pts',(-2.75,-16.9270123243332,41.4317871928215));
#13686=CARTESIAN_POINT('Ctrl Pts',(-3.,-16.4822646677494,41.7046384811401));
#13687=CARTESIAN_POINT('Ctrl Pts',(-2.75,-16.4822646677494,41.7046384811401));
#13688=CARTESIAN_POINT('',(-2.75,-17.4918144643307,41.4317871928215));
#13689=CARTESIAN_POINT('',(-3.,-17.4918144643307,41.4317871928215));
#13690=CARTESIAN_POINT('',(-2.75,-16.4822646677494,41.7046384811401));
#13691=CARTESIAN_POINT('Ctrl Pts',(-2.75,-17.4918144643307,41.4317871928215));
#13692=CARTESIAN_POINT('Ctrl Pts',(-2.75,-16.9270123243332,41.4317871928215));
#13693=CARTESIAN_POINT('Ctrl Pts',(-2.75,-16.4822646677494,41.7046384811401));
#13694=CARTESIAN_POINT('',(-3.,-16.4822646677494,41.7046384811401));
#13695=CARTESIAN_POINT('Ctrl Pts',(-3.,-18.4631651341915,41.6787176132202));
#13696=CARTESIAN_POINT('Ctrl Pts',(-2.75,-18.4631651341915,41.6787176132202));
#13697=CARTESIAN_POINT('Ctrl Pts',(-3.,-18.0129605233669,41.4317871928215));
#13698=CARTESIAN_POINT('Ctrl Pts',(-2.75,-18.0129605233669,41.4317871928215));
#13699=CARTESIAN_POINT('Ctrl Pts',(-3.,-17.4918144643307,41.4317871928215));
#13700=CARTESIAN_POINT('Ctrl Pts',(-2.75,-17.4918144643307,41.4317871928215));
#13701=CARTESIAN_POINT('',(-2.75,-18.4631651341915,41.6787176132202));
#13702=CARTESIAN_POINT('',(-3.,-18.4631651341915,41.6787176132202));
#13703=CARTESIAN_POINT('Ctrl Pts',(-2.75,-18.4631651341915,41.6787176132202));
#13704=CARTESIAN_POINT('Ctrl Pts',(-2.75,-18.0129605233669,41.4317871928215));
#13705=CARTESIAN_POINT('Ctrl Pts',(-2.75,-17.4918144643307,41.4317871928215));
#13706=CARTESIAN_POINT('Ctrl Pts',(-3.,-19.1589361131191,42.4058662652969));
#13707=CARTESIAN_POINT('Ctrl Pts',(-2.75,-19.1589361131191,42.4058662652969));
#13708=CARTESIAN_POINT('Ctrl Pts',(-3.,-18.9133697450161,41.9256480336189));
#13709=CARTESIAN_POINT('Ctrl Pts',(-2.75,-18.9133697450161,41.9256480336189));
#13710=CARTESIAN_POINT('Ctrl Pts',(-3.,-18.4631651341915,41.6787176132202));
#13711=CARTESIAN_POINT('Ctrl Pts',(-2.75,-18.4631651341915,41.6787176132202));
#13712=CARTESIAN_POINT('',(-2.75,-19.1589361131191,42.4058662652969));
#13713=CARTESIAN_POINT('',(-3.,-19.1589361131191,42.4058662652969));
#13714=CARTESIAN_POINT('Ctrl Pts',(-2.75,-19.1589361131191,42.4058662652969));
#13715=CARTESIAN_POINT('Ctrl Pts',(-2.75,-18.9133697450161,41.9256480336189));
#13716=CARTESIAN_POINT('Ctrl Pts',(-2.75,-18.4631651341915,41.6787176132202));
#13717=CARTESIAN_POINT('Ctrl Pts',(-3.,-19.4045021831989,43.4945430159569));
#13718=CARTESIAN_POINT('Ctrl Pts',(-2.75,-19.4045021831989,43.4945430159569));
#13719=CARTESIAN_POINT('Ctrl Pts',(-3.,-19.4045021831989,42.8860844969749));
#13720=CARTESIAN_POINT('Ctrl Pts',(-2.75,-19.4045021831989,42.8860844969749));
#13721=CARTESIAN_POINT('Ctrl Pts',(-3.,-19.1589361131191,42.4058662652969));
#13722=CARTESIAN_POINT('Ctrl Pts',(-2.75,-19.1589361131191,42.4058662652969));
#13723=CARTESIAN_POINT('',(-2.75,-19.4045021831989,43.4945430159569));
#13724=CARTESIAN_POINT('',(-3.,-19.4045021831989,43.4945430159569));
#13725=CARTESIAN_POINT('Ctrl Pts',(-2.75,-19.4045021831989,43.4945430159569));
#13726=CARTESIAN_POINT('Ctrl Pts',(-2.75,-19.4045021831989,42.8860844969749));
#13727=CARTESIAN_POINT('Ctrl Pts',(-2.75,-19.1589361131191,42.4058662652969));
#13728=CARTESIAN_POINT('Ctrl Pts',(-3.,-19.1712143719196,44.5682128071785));
#13729=CARTESIAN_POINT('Ctrl Pts',(-2.75,-19.1712143719196,44.5682128071785));
#13730=CARTESIAN_POINT('Ctrl Pts',(-3.,-19.4045021831989,44.0948157310486));
#13731=CARTESIAN_POINT('Ctrl Pts',(-2.75,-19.4045021831989,44.0948157310486));
#13732=CARTESIAN_POINT('Ctrl Pts',(-3.,-19.4045021831989,43.4945430159569));
#13733=CARTESIAN_POINT('Ctrl Pts',(-2.75,-19.4045021831989,43.4945430159569));
#13734=CARTESIAN_POINT('',(-2.75,-19.1712143719196,44.5682128071785));
#13735=CARTESIAN_POINT('',(-3.,-19.1712143719196,44.5682128071785));
#13736=CARTESIAN_POINT('Ctrl Pts',(-2.75,-19.1712143719196,44.5682128071785));
#13737=CARTESIAN_POINT('Ctrl Pts',(-2.75,-19.4045021831989,44.0948157310486));
#13738=CARTESIAN_POINT('Ctrl Pts',(-2.75,-19.4045021831989,43.4945430159569));
#13739=CARTESIAN_POINT('Ctrl Pts',(-3.,-18.4931787550449,45.30627566576));
#13740=CARTESIAN_POINT('Ctrl Pts',(-2.75,-18.4931787550449,45.30627566576));
#13741=CARTESIAN_POINT('Ctrl Pts',(-3.,-18.9379265606403,45.0416098833084));
#13742=CARTESIAN_POINT('Ctrl Pts',(-2.75,-18.9379265606403,45.0416098833084));
#13743=CARTESIAN_POINT('Ctrl Pts',(-3.,-19.1712143719196,44.5682128071785));
#13744=CARTESIAN_POINT('Ctrl Pts',(-2.75,-19.1712143719196,44.5682128071785));
#13745=CARTESIAN_POINT('',(-2.75,-18.4931787550449,45.30627566576));
#13746=CARTESIAN_POINT('',(-3.,-18.4931787550449,45.30627566576));
#13747=CARTESIAN_POINT('Ctrl Pts',(-2.75,-18.4931787550449,45.30627566576));
#13748=CARTESIAN_POINT('Ctrl Pts',(-2.75,-18.9379265606403,45.0416098833084));
#13749=CARTESIAN_POINT('Ctrl Pts',(-2.75,-19.1712143719196,44.5682128071785));
#13750=CARTESIAN_POINT('Ctrl Pts',(-3.,-17.4945430159569,45.5709411501884));
#13751=CARTESIAN_POINT('Ctrl Pts',(-2.75,-17.4945430159569,45.5709411501884));
#13752=CARTESIAN_POINT('Ctrl Pts',(-3.,-18.0484312474728,45.5709411501884));
#13753=CARTESIAN_POINT('Ctrl Pts',(-2.75,-18.0484312474728,45.5709411501884));
#13754=CARTESIAN_POINT('Ctrl Pts',(-3.,-18.4931787550449,45.30627566576));
#13755=CARTESIAN_POINT('Ctrl Pts',(-2.75,-18.4931787550449,45.30627566576));
#13756=CARTESIAN_POINT('',(-2.75,-17.4945430159569,45.5709411501884));
#13757=CARTESIAN_POINT('',(-3.,-17.4945430159569,45.5709411501884));
#13758=CARTESIAN_POINT('Ctrl Pts',(-2.75,-17.4945430159569,45.5709411501884));
#13759=CARTESIAN_POINT('Ctrl Pts',(-2.75,-18.0484312474728,45.5709411501884));
#13760=CARTESIAN_POINT('Ctrl Pts',(-2.75,-18.4931787550449,45.30627566576));
#13761=CARTESIAN_POINT('Ctrl Pts',(-3.,-16.1139154136181,45.0075035095215));
#13762=CARTESIAN_POINT('Ctrl Pts',(-2.75,-16.1139154136181,45.0075035095215));
#13763=CARTESIAN_POINT('Ctrl Pts',(-3.,-16.6487039327621,45.5709411501884));
#13764=CARTESIAN_POINT('Ctrl Pts',(-2.75,-16.6487039327621,45.5709411501884));
#13765=CARTESIAN_POINT('Ctrl Pts',(-3.,-17.4945430159569,45.5709411501884));
#13766=CARTESIAN_POINT('Ctrl Pts',(-2.75,-17.4945430159569,45.5709411501884));
#13767=CARTESIAN_POINT('',(-2.75,-16.1139154136181,45.0075035095215));
#13768=CARTESIAN_POINT('',(-3.,-16.1139154136181,45.0075035095215));
#13769=CARTESIAN_POINT('Ctrl Pts',(-2.75,-16.1139154136181,45.0075035095215));
#13770=CARTESIAN_POINT('Ctrl Pts',(-2.75,-16.6487039327621,45.5709411501884));
#13771=CARTESIAN_POINT('Ctrl Pts',(-2.75,-17.4945430159569,45.5709411501884));
#13772=CARTESIAN_POINT('Ctrl Pts',(-3.,-15.5791269317269,43.4481580853462));
#13773=CARTESIAN_POINT('Ctrl Pts',(-2.75,-15.5791269317269,43.4481580853462));
#13774=CARTESIAN_POINT('Ctrl Pts',(-3.,-15.5791269317269,44.4440655708313));
#13775=CARTESIAN_POINT('Ctrl Pts',(-2.75,-15.5791269317269,44.4440655708313));
#13776=CARTESIAN_POINT('Ctrl Pts',(-3.,-16.1139154136181,45.0075035095215));
#13777=CARTESIAN_POINT('Ctrl Pts',(-2.75,-16.1139154136181,45.0075035095215));
#13778=CARTESIAN_POINT('',(-2.75,-15.5791269317269,43.4481580853462));
#13779=CARTESIAN_POINT('',(-3.,-15.5791269317269,43.4481580853462));
#13780=CARTESIAN_POINT('Ctrl Pts',(-2.75,-15.5791269317269,43.4481580853462));
#13781=CARTESIAN_POINT('Ctrl Pts',(-2.75,-15.5791269317269,44.4440655708313));
#13782=CARTESIAN_POINT('Ctrl Pts',(-2.75,-16.1139154136181,45.0075035095215));
#13783=CARTESIAN_POINT('Ctrl Pts',(-3.,-15.8083220273256,42.4495224952698));
#13784=CARTESIAN_POINT('Ctrl Pts',(-2.75,-15.8083220273256,42.4495224952698));
#13785=CARTESIAN_POINT('Ctrl Pts',(-3.,-15.5791269317269,42.9215552210808));
#13786=CARTESIAN_POINT('Ctrl Pts',(-2.75,-15.5791269317269,42.9215552210808));
#13787=CARTESIAN_POINT('Ctrl Pts',(-3.,-15.5791269317269,43.4481580853462));
#13788=CARTESIAN_POINT('Ctrl Pts',(-2.75,-15.5791269317269,43.4481580853462));
#13789=CARTESIAN_POINT('',(-2.75,-15.8083220273256,42.4495224952698));
#13790=CARTESIAN_POINT('',(-3.,-15.8083220273256,42.4495224952698));
#13791=CARTESIAN_POINT('Ctrl Pts',(-2.75,-15.8083220273256,42.4495224952698));
#13792=CARTESIAN_POINT('Ctrl Pts',(-2.75,-15.5791269317269,42.9215552210808));
#13793=CARTESIAN_POINT('Ctrl Pts',(-2.75,-15.5791269317269,43.4481580853462));
#13794=CARTESIAN_POINT('Ctrl Pts',(-3.,-16.4822646677494,41.7046384811401));
#13795=CARTESIAN_POINT('Ctrl Pts',(-2.75,-16.4822646677494,41.7046384811401));
#13796=CARTESIAN_POINT('Ctrl Pts',(-3.,-16.0375170856714,41.9774897694588));
#13797=CARTESIAN_POINT('Ctrl Pts',(-2.75,-16.0375170856714,41.9774897694588));
#13798=CARTESIAN_POINT('Ctrl Pts',(-3.,-15.8083220273256,42.4495224952698));
#13799=CARTESIAN_POINT('Ctrl Pts',(-2.75,-15.8083220273256,42.4495224952698));
#13800=CARTESIAN_POINT('Ctrl Pts',(-2.75,-16.4822646677494,41.7046384811401));
#13801=CARTESIAN_POINT('Ctrl Pts',(-2.75,-16.0375170856714,41.9774897694588));
#13802=CARTESIAN_POINT('Ctrl Pts',(-2.75,-15.8083220273256,42.4495224952698));
#13803=CARTESIAN_POINT('Origin',(-2.75,-17.4918145574629,43.501364171505));
#13804=CARTESIAN_POINT('Origin',(-3.,25.,66.5));
#13805=CARTESIAN_POINT('',(-3.,25.,68.2));
#13806=CARTESIAN_POINT('Origin',(-3.,-25.,26.5));
#13807=CARTESIAN_POINT('',(-3.,-25.,28.2));
#13808=CARTESIAN_POINT('Origin',(-3.,-25.,66.5));
#13809=CARTESIAN_POINT('',(-3.,-25.,68.2));
#13810=CARTESIAN_POINT('Origin',(-3.,25.,26.5));
#13811=CARTESIAN_POINT('',(-3.,25.,28.2));
#13812=CARTESIAN_POINT('Origin',(-3.,0.,47.5));
#13813=CARTESIAN_POINT('',(-3.,-7.9602041944578E-16,54.));
#13814=CARTESIAN_POINT('Origin',(0.,25.1,26.5));
#13815=CARTESIAN_POINT('',(0.,25.1,22.5));
#13816=CARTESIAN_POINT('Origin',(0.,-25.1,26.5));
#13817=CARTESIAN_POINT('',(0.,-25.1,22.5));
#13818=CARTESIAN_POINT('Origin',(0.,29.1,22.5));
#18255=UNCERTAINTY_MEASURE_WITH_UNIT(LENGTH_MEASURE(0.01),#18282,
'DISTANCE_ACCURACY_VALUE',
'Maximum model space distance between geometric entities at asserted c
onnectivities');
#18266=UNCERTAINTY_MEASURE_WITH_UNIT(LENGTH_MEASURE(0.01),#18282,
'DISTANCE_ACCURACY_VALUE',
'Maximum model space distance between geometric entities at asserted c
onnectivities');
#18270=(
GEOMETRIC_REPRESENTATION_CONTEXT(3)
GLOBAL_UNCERTAINTY_ASSIGNED_CONTEXT((#18255))
GLOBAL_UNIT_ASSIGNED_CONTEXT((#18282,#18284,#18285))
REPRESENTATION_CONTEXT('','3D')
);
#18281=(
GEOMETRIC_REPRESENTATION_CONTEXT(3)
GLOBAL_UNCERTAINTY_ASSIGNED_CONTEXT((#18266))
GLOBAL_UNIT_ASSIGNED_CONTEXT((#18282,#18284,#18285))
REPRESENTATION_CONTEXT('','3D')
);
#18282=(
LENGTH_UNIT()
NAMED_UNIT(*)
SI_UNIT(.MILLI.,.METRE.)
);
#18284=(
NAMED_UNIT(*)
PLANE_ANGLE_UNIT()
SI_UNIT($,.RADIAN.)
);
#18285=(
NAMED_UNIT(*)
SI_UNIT($,.STERADIAN.)
SOLID_ANGLE_UNIT()
);
#18289=SHAPE_DEFINITION_REPRESENTATION(#18303,#18341);
#18303=PRODUCT_DEFINITION_SHAPE('',$,#18356);
#18341=SHAPE_REPRESENTATION('',(#9302),#18270);
#18352=PRODUCT_DEFINITION_CONTEXT('part definition',#18396,'design');
#18356=PRODUCT_DEFINITION('2026-10-20-13-03-18-998',
'06_Front_Label_Plate_ON-OFF',#18370,#18352);
#18370=PRODUCT_DEFINITION_FORMATION('',$,#18401);
#18396=APPLICATION_CONTEXT(
'Core Data for Automotive Mechanical Design Process');
#18397=PRODUCT_CONTEXT('part definition',#18396,'mechanical');
#18401=PRODUCT('2026-10-20-13-03-18-998','06_Front_Label_Plate_ON-OFF',
$,(#18397));
#18482=COLOUR_RGB('Off White',0.89,0.88,0.83);
#18483=FILL_AREA_STYLE_COLOUR('',#18482);
#18484=FILL_AREA_STYLE('',(#18483));
#18485=SURFACE_STYLE_FILL_AREA(#18484);
#18486=SURFACE_SIDE_STYLE('',(#18485));
#18487=SURFACE_STYLE_USAGE(.BOTH.,#18486);
#18488=PRESENTATION_STYLE_ASSIGNMENT((#18487));
ENDSEC;
END-ISO-10303-21;
